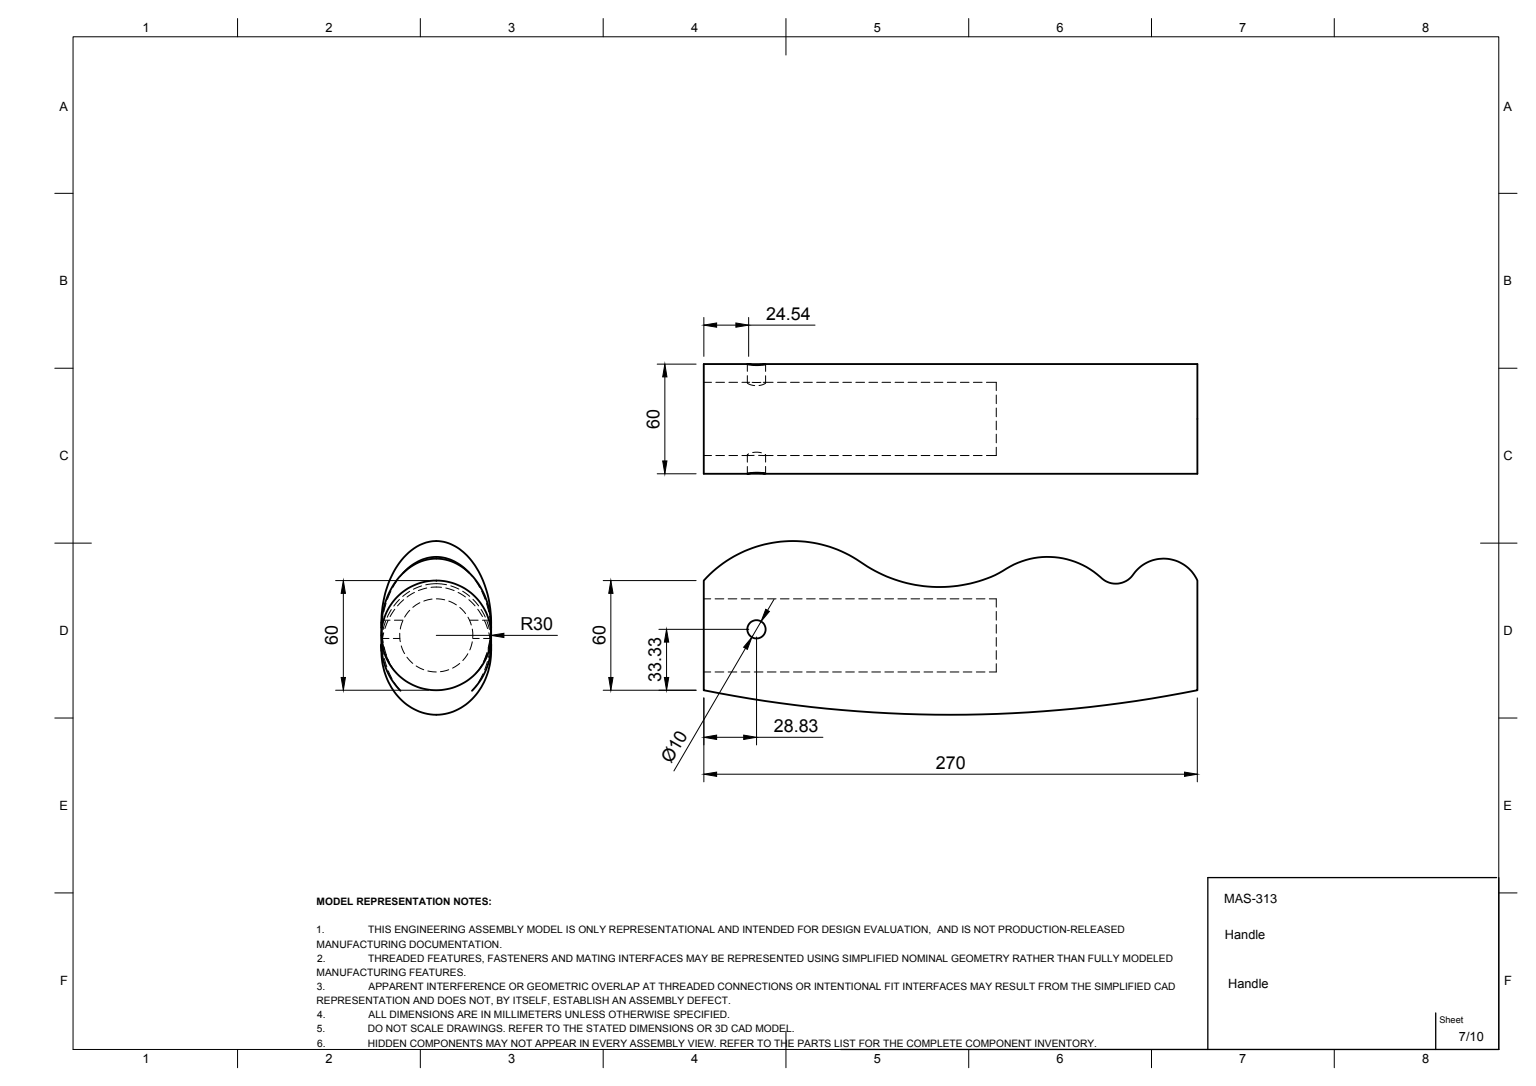
ISO-10303-21;
HEADER;
FILE_DESCRIPTION (('STEP AP214'),
    '1' );
FILE_NAME ('Handle.step',
    '2026-10-06T09:36:00',
    ( '' ),
    ( '' ),
    'SwSTEP 2.0',
    'SolidWorks 2025',
    '' );
FILE_SCHEMA (( 'AUTOMOTIVE_DESIGN' ));
ENDSEC;

DATA;
#4=CARTESIAN_POINT ( 'NONE',  ( -828.8285638327245124, 78.34605190446923473, -105.0145692953451260 ) ) ;
#15=CARTESIAN_POINT ( 'NONE',  ( -795.0000000000070486, 70.44548139156158584, -96.78565065507937959 ) ) ;
#16=CARTESIAN_POINT ( 'NONE',  ( -820.7717470982067880, 82.64484858469236883, -104.6903222377189593 ) ) ;
#19=CARTESIAN_POINT ( 'NONE',  ( -826.0529305544633871, 83.16438776978758085, -144.6472496521801929 ) ) ;
#28=CARTESIAN_POINT ( 'NONE',  ( -976.0610374937461984, 42.74778062430068104, -107.9061927053324155 ) ) ;
#38=CARTESIAN_POINT ( 'NONE',  ( -795.0000000000065938, 109.8950841424301217, -113.1262384684096105 ) ) ;
#41=CARTESIAN_POINT ( 'NONE',  ( -951.5459139781262365, 122.3346817490816676, -136.2353035311979852 ) ) ;
#50=CARTESIAN_POINT ( 'NONE',  ( -954.3284336448712111, 118.5422944683825932, -141.4553492942762318 ) ) ;
#59=CARTESIAN_POINT ( 'NONE',  ( -1046.457602311632627, 98.67849639484583690, -149.7857175106632894 ) ) ;
#60=CARTESIAN_POINT ( 'NONE',  ( -1054.407929976944160, 113.5897173251037628, -130.5712005305405228 ) ) ;
#67=CARTESIAN_POINT ( 'NONE',  ( -1027.708477481189902, 65.70736702952426356, -149.7857175106639431 ) ) ;
#79=CARTESIAN_POINT ( 'NONE',  ( -1062.665377791213132, 57.01990411978262330, -103.3307627799634503 ) ) ;
#82=CARTESIAN_POINT ( 'NONE',  ( -1032.658196452833636, 44.72920460984212809, -126.6442663926291914 ) ) ;
#91=CARTESIAN_POINT ( 'NONE',  ( -953.8433812051914629, 65.95343150956773570, -99.57582448894520155 ) ) ;
#98=CARTESIAN_POINT ( 'NONE',  ( -1054.691024341069351, 108.1159421897237110, -107.9061927053325149 ) ) ;
#104=CARTESIAN_POINT ( 'NONE',  ( -1054.519145619997744, 111.4921997120089401, -113.1262384684101079 ) ) ;
#107=CARTESIAN_POINT ( 'NONE',  ( -1024.848917040341576, 116.4131098345822437, -136.2353035311980420 ) ) ;
#109=CARTESIAN_POINT ( 'NONE',  ( -1045.884592419585942, 115.0579440276405450, -118.7903414690682524 ) ) ;
#113=CARTESIAN_POINT ( 'NONE',  ( -954.7734463792789938, 107.7731650919854758, -149.7857175106632042 ) ) ;
#119=CARTESIAN_POINT ( 'NONE',  ( -1065.000000000006366, 107.1049510380562850, -141.4553492942759192 ) ) ;
#129=CARTESIAN_POINT ( 'NONE',  ( -956.7203770923184720, 58.97922774997713447, -146.0307792196449839 ) ) ;
#137=CARTESIAN_POINT ( 'NONE',  ( -818.1708872189576596, 40.82851623284144438, -103.3307627799635640 ) ) ;
#138=CARTESIAN_POINT ( 'NONE',  ( -823.5000624989293101, 83.67424195610622917, -104.7509713550767287 ) ) ;
#139=CARTESIAN_POINT ( 'NONE',  ( -901.8967518049312275, 57.00804855647886171, -130.5712005305400965 ) ) ;
#140=VERTEX_POINT ( 'NONE', #3194 ) ;
#142=CARTESIAN_POINT ( 'NONE',  ( -825.4378685752795946, 73.92905737501402541, -154.6600603160834169 ) ) ;
#146=CARTESIAN_POINT ( 'NONE',  ( -1021.607260580486013, 54.24386729702176524, -118.7903414690683661 ) ) ;
#155=CARTESIAN_POINT ( 'NONE',  ( -954.3284336448667773, 118.5422944683823800, -107.9061927053323302 ) ) ;
#158=CARTESIAN_POINT ( 'NONE',  ( -1054.519145619990923, 111.4921997120091106, -136.2353035311978999 ) ) ;
#169=CARTESIAN_POINT ( 'NONE',  ( -852.9318753287220716, 113.3383058689776277, -141.4553492942764024 ) ) ;
#178=VERTEX_POINT ( 'NONE', #3366 ) ;
#182=CARTESIAN_POINT ( 'NONE',  ( -956.4793285278399253, 64.87563161486532692, -149.7857175106635452 ) ) ;
#190=CARTESIAN_POINT ( 'NONE',  ( -954.4431216459919369, 51.77564274757662588, -136.2353035311985820 ) ) ;
#194=CARTESIAN_POINT ( 'NONE',  ( -817.4144546772188278, 30.82543593413045713, -113.1262384684093689 ) ) ;
#195=CARTESIAN_POINT ( 'NONE',  ( -822.2163178171820164, 83.41010758653678181, -104.7304854148475499 ) ) ;
#202=CARTESIAN_POINT ( 'NONE',  ( -828.1602791247941013, 76.17169011767150266, -154.6744596958750151 ) ) ;
#207=CARTESIAN_POINT ( 'NONE',  ( -1048.438004920983758, 39.66697241395321782, -122.7172756069793138 ) ) ;
#212=UNCERTAINTY_MEASURE_WITH_UNIT (LENGTH_MEASURE( 1.000000000000000082E-05 ), #7205, 'distance_accuracy_value', 'NONE');
#214=CARTESIAN_POINT ( 'NONE',  ( -951.5459139781289650, 122.3346817490815681, -113.1262384684093263 ) ) ;
#219=CARTESIAN_POINT ( 'NONE',  ( -1061.673215548682720, 86.58918783539685649, -95.06748246948023962 ) ) ;
#220=CARTESIAN_POINT ( 'NONE',  ( -954.0688428831344936, 124.4732772249357282, -130.5712005305405796 ) ) ;
#229=CARTESIAN_POINT ( 'NONE',  ( -1025.044148074459827, 113.2108726315406813, -141.4553492942762318 ) ) ;
#234=CARTESIAN_POINT ( 'NONE',  ( -1010.922847972424620, 120.6260792194949829, -126.6442663926288503 ) ) ;
#237=CARTESIAN_POINT ( 'NONE',  ( -853.1108559448500728, 99.60875591605696400, -149.7857175106632610 ) ) ;
#245=CARTESIAN_POINT ( 'NONE',  ( -956.2104666674752025, 71.56905446038098262, -152.5758913445294809 ) ) ;
#251=CARTESIAN_POINT ( 'NONE',  ( -795.0000000000020464, 52.38665522077208436, -130.5712005305402670 ) ) ;
#252=ORIENTED_EDGE ( 'NONE', *, *, #941, .T. ) ;
#257=CARTESIAN_POINT ( 'NONE',  ( -1014.004070199759440, 54.58258344709550869, -113.1262384684095537 ) ) ;
#259=CARTESIAN_POINT ( 'NONE',  ( -1014.004070199769671, 54.58258344709567922, -136.2353035311988947 ) ) ;
#265=CARTESIAN_POINT ( 'NONE',  ( -976.2351830775012331, 35.86345807843999012, -118.7903414690679824 ) ) ;
#272=CARTESIAN_POINT ( 'NONE',  ( -1031.197907781702725, 107.2697845108577894, -103.3307627799635640 ) ) ;
#279=DIRECTION ( 'NONE',  ( 1.000000000000000000, -1.262554838833776231E-16, 0.000000000000000000 ) ) ;
#282=CARTESIAN_POINT ( 'NONE',  ( -853.3345817150102448, 81.97571759610518427, -95.06748246948041015 ) ) ;
#284=CARTESIAN_POINT ( 'NONE',  ( -823.5047064235034213, 114.4566975831562274, -136.2353035311979284 ) ) ;
#293=CARTESIAN_POINT ( 'NONE',  ( -1037.392967692951970, 114.2240391150264998, -136.2353035311982126 ) ) ;
#300=CARTESIAN_POINT ( 'NONE',  ( -1060.756016675586807, 112.8516620848305934, -124.6807709998040821 ) ) ;
#302=CARTESIAN_POINT ( 'NONE',  ( -1037.550865396555764, 105.7975851359348667, -146.0307792196445860 ) ) ;
#309=CARTESIAN_POINT ( 'NONE',  ( -953.8433812051875975, 65.95343150956774991, -149.7857175106634315 ) ) ;
#313=CARTESIAN_POINT ( 'NONE',  ( -854.0803342822151762, 23.97549884981696167, -130.5712005305403238 ) ) ;
#317=CARTESIAN_POINT ( 'NONE',  ( -1028.454949082212806, 53.01113643315385104, -113.1262384684094400 ) ) ;
#320=CARTESIAN_POINT ( 'NONE',  ( -1038.664246639927342, 43.28664065472985811, -136.2353035311990084 ) ) ;
#326=CARTESIAN_POINT ( 'NONE',  ( -824.4849247483655290, 73.70682285379986354, -154.6506428397234743 ) ) ;
#329=CARTESIAN_POINT ( 'NONE',  ( -1065.000000000003865, 52.00000000000021316, -126.6442663926290493 ) ) ;
#335=CARTESIAN_POINT ( 'NONE',  ( -1061.468168685228193, 92.73456844357777129, -96.78565065507918064 ) ) ;
#341=CIRCLE ( 'NONE', #6268, 30.00000000000021316 ) ;
#345=CARTESIAN_POINT ( 'NONE',  ( -1055.782959745578182, 85.17781532426863578, -95.06748246948041015 ) ) ;
#347=CARTESIAN_POINT ( 'NONE',  ( -1021.743962174751232, 119.2557508373789403, -124.6807709998040110 ) ) ;
#354=CARTESIAN_POINT ( 'NONE',  ( -1048.438004920983303, 39.66697241395321782, -124.6807709998044800 ) ) ;
#360=PLANE ( 'NONE',  #530 ) ;
#361=CARTESIAN_POINT ( 'NONE',  ( -1024.691966601151762, 118.8493250655917564, -126.6442663926291061 ) ) ;
#374=CARTESIAN_POINT ( 'NONE',  ( -827.5978224575839022, 75.37295367873073815, -94.68020981275554959 ) ) ;
#375=( NAMED_UNIT ( * ) SI_UNIT ( $, .STERADIAN. ) SOLID_ANGLE_UNIT ( ) );
#378=CARTESIAN_POINT ( 'NONE',  ( -1062.923339974281134, 49.86928741160674150, -136.2353035311989515 ) ) ;
#382=CARTESIAN_POINT ( 'NONE',  ( -1017.158871447982051, 53.64146012065780411, -122.7172756069791717 ) ) ;
#385=CARTESIAN_POINT ( 'NONE',  ( -822.5313098515729280, 73.83434793536794416, -154.6477719089843390 ) ) ;
#388=CARTESIAN_POINT ( 'NONE',  ( -976.2517683711888594, 35.25052392388814582, -122.7172756069790296 ) ) ;
#393=CARTESIAN_POINT ( 'NONE',  ( -1025.928429817214464, 97.79385104913474436, -96.78565065507955012 ) ) ;
#397=CARTESIAN_POINT ( 'NONE',  ( -795.0000000000002274, 98.77454568802498613, -99.57582448894500260 ) ) ;
#399=CARTESIAN_POINT ( 'NONE',  ( -951.4198147059589701, 125.0824040815807194, -124.6807709998040252 ) ) ;
#410=CARTESIAN_POINT ( 'NONE',  ( -1017.810720698608179, 119.7719591276206046, -126.6442663926290493 ) ) ;
#415=ORIENTED_EDGE ( 'NONE', *, *, #2463, .T. ) ;
#425=CARTESIAN_POINT ( 'NONE',  ( -901.9718911164696920, 59.00785292138922244, -136.2353035311984115 ) ) ;
#430=CARTESIAN_POINT ( 'NONE',  ( -1062.996098538733122, 47.98024286075321498, -118.7903414690683377 ) ) ;
#432=CARTESIAN_POINT ( 'NONE',  ( -824.1522960622456822, 83.67452213711085562, -95.25851046848316628 ) ) ;
#433=CARTESIAN_POINT ( 'NONE',  ( -818.8285638327243987, 78.67432280806558254, -94.73795703228648790 ) ) ;
#437=CARTESIAN_POINT ( 'NONE',  ( -1021.637154595298057, 53.81063926482157456, -126.6442663926291630 ) ) ;
#439=CARTESIAN_POINT ( 'NONE',  ( -818.8285638327238303, 78.67432280806571043, -144.4023295390032899 ) ) ;
#443=CARTESIAN_POINT ( 'NONE',  ( -1031.329434936836833, 101.6864263019767378, -99.57582448894520155 ) ) ;
#453=CARTESIAN_POINT ( 'NONE',  ( -828.7969121913764639, 79.32510138126919230, -154.5423082524717699 ) ) ;
#454=CARTESIAN_POINT ( 'NONE',  ( -1038.158164256576356, 71.32123499372119113, -95.06748246948035330 ) ) ;
#456=CARTESIAN_POINT ( 'NONE',  ( -823.7180591916866206, 117.1502831467254993, -130.5712005305406080 ) ) ;
#464=CARTESIAN_POINT ( 'NONE',  ( -795.0000000000020464, 111.6133447792289530, -118.7903414690682524 ) ) ;
#467=CARTESIAN_POINT ( 'NONE',  ( -795.0000000000048885, 52.00000000000024158, -124.6807709998040821 ) ) ;
#477=CARTESIAN_POINT ( 'NONE',  ( -955.0000000000038654, 102.0000000000005400, -124.6807709998041531 ) ) ;
#480=EDGE_LOOP ( 'NONE', ( #1423, #3316 ) ) ;
#485=CARTESIAN_POINT ( 'NONE',  ( -902.6139906877482417, 77.75433758651681160, -152.5758913445294809 ) ) ;
#486=CARTESIAN_POINT ( 'NONE',  ( -818.9962482452939412, 77.37998253221861944, -144.1405054422210981 ) ) ;
#494=CARTESIAN_POINT ( 'NONE',  ( -1013.844210246968942, 57.79547239392000790, -141.4553492942758908 ) ) ;
#499=CARTESIAN_POINT ( 'NONE',  ( -827.5988398165042099, 81.97491382366440860, -95.05718603569194158 ) ) ;
#506=CARTESIAN_POINT ( 'NONE',  ( -998.0431609429218724, 37.14019503514174403, -126.6442663926292340 ) ) ;
#512=CARTESIAN_POINT ( 'NONE',  ( -974.6181169426257611, 104.3135445892214506, -99.57582448894483207 ) ) ;
#523=CARTESIAN_POINT ( 'NONE',  ( -903.0443340174317655, 90.92133391050421665, -94.48732055948569553 ) ) ;
#526=CARTESIAN_POINT ( 'NONE',  ( -1017.810720698608179, 119.7719591276206046, -126.6442663926290493 ) ) ;
#530=AXIS2_PLACEMENT_3D ( 'NONE', #4144, #3201, #7285 ) ;
#535=CARTESIAN_POINT ( 'NONE',  ( -823.4987033863208126, 83.67412160126858112, -95.25369430085760314 ) ) ;
#538=CARTESIAN_POINT ( 'NONE',  ( -904.2101318206010774, 125.2895275102983419, -122.7172756069790580 ) ) ;
#557=CARTESIAN_POINT ( 'NONE',  ( -824.4876953351460998, 73.70726043279957196, -94.71087641695557124 ) ) ;
#561=CARTESIAN_POINT ( 'NONE',  ( -927.9936929689694125, 74.21188826700395680, -149.7857175106638863 ) ) ;
#570=CARTESIAN_POINT ( 'NONE',  ( -828.7958589970872936, 79.33211491968606310, -94.81972313272032693 ) ) ;
#575=CARTESIAN_POINT ( 'NONE',  ( -955.0000000000038654, 82.00000000000036948, -124.6807709998041673 ) ) ;
#581=CARTESIAN_POINT ( 'NONE',  ( -994.8066578865433485, 80.00401887192406036, -94.48732055948607922 ) ) ;
#592=CARTESIAN_POINT ( 'NONE',  ( -826.3386627754631490, 83.01093823284401196, -154.1821612695491979 ) ) ;
#593=CARTESIAN_POINT ( 'NONE',  ( -902.6139906877451722, 77.75433758651645633, -96.78565065507919485 ) ) ;
#600=CARTESIAN_POINT ( 'NONE',  ( -817.1493800258449482, 27.50875274330016751, -124.6807709998041815 ) ) ;
#602=FACE_OUTER_BOUND ( 'NONE', #11018, .T. ) ;
#603=CARTESIAN_POINT ( 'NONE',  ( -1037.337636019038655, 116.9882293220588991, -122.7172756069792001 ) ) ;
#614=CARTESIAN_POINT ( 'NONE',  ( -1020.082665824768128, 80.34198733739798115, -154.2940595301280950 ) ) ;
#624=ORIENTED_EDGE ( 'NONE', *, *, #2970, .T. ) ;
#625=CARTESIAN_POINT ( 'NONE',  ( -976.0610374937396045, 42.74778062430040393, -141.4553492942756634 ) ) ;
#643=CARTESIAN_POINT ( 'NONE',  ( -1065.000000000006139, 76.10956187831460795, -95.06748246948023962 ) ) ;
#653=CARTESIAN_POINT ( 'NONE',  ( -1012.828629370415570, 79.69572830938430741, -95.06748246948046699 ) ) ;
#668=CARTESIAN_POINT ( 'NONE',  ( -1065.000000000007731, 112.0000000000007105, -122.7172756069790438 ) ) ;
#673=AXIS2_PLACEMENT_3D ( 'NONE', #5309, #8235, #11995 ) ;
#679=CARTESIAN_POINT ( 'NONE',  ( -1061.673215548682947, 86.58918783539726860, -154.2940595301283793 ) ) ;
#684=CARTESIAN_POINT ( 'NONE',  ( -1014.911393615049064, 99.73439156315002663, -152.5758913445290261 ) ) ;
#689=CARTESIAN_POINT ( 'NONE',  ( -1065.000000000003638, 87.89043812168645786, -154.2940595301284361 ) ) ;
#702=CARTESIAN_POINT ( 'NONE',  ( -1065.000000000000682, 52.38665522077219805, -130.5712005305403238 ) ) ;
#717=CARTESIAN_POINT ( 'NONE',  ( -853.5732225365160275, 62.99598188221410311, -95.06748246948041015 ) ) ;
#718=PLANE ( 'NONE',  #10433 ) ;
#732=CARTESIAN_POINT ( 'NONE',  ( -1017.810720698610226, 119.7719591276204625, -122.7172756069789017 ) ) ;
#743=CARTESIAN_POINT ( 'NONE',  ( -994.8066578865465317, 80.00401887192411721, -154.8742214401228523 ) ) ;
#744=CARTESIAN_POINT ( 'NONE',  ( -828.5731535248166892, 77.06390383656801646, -144.0645491675088294 ) ) ;
#747=CARTESIAN_POINT ( 'NONE',  ( -794.9999999999980673, 87.89043812168634418, -154.2940595301278961 ) ) ;
#751=STYLED_ITEM ( 'NONE', ( #7990 ), #8008 ) ;
#754=CARTESIAN_POINT ( 'NONE',  ( -1065.000000000004320, 98.77454568802519930, -149.7857175106631189 ) ) ;
#756=CARTESIAN_POINT ( 'NONE',  ( -1047.392513188124212, 70.23666496464454667, -154.2940595301285214 ) ) ;
#764=CARTESIAN_POINT ( 'NONE',  ( -817.4144546772251942, 30.82543593413060279, -136.2353035311987242 ) ) ;
#776=CARTESIAN_POINT ( 'NONE',  ( -995.4135022096149896, 71.70161378084165449, -95.06748246948046699 ) ) ;
#779=CARTESIAN_POINT ( 'NONE',  ( -820.7807412222841776, 82.64141399635654750, -144.6707558958804043 ) ) ;
#788=CARTESIAN_POINT ( 'NONE',  ( -1062.665377791213132, 57.01990411978262330, -103.3307627799634503 ) ) ;
#803=CARTESIAN_POINT ( 'NONE',  ( -1021.777026427247165, 118.8177985574657924, -118.7903414690675561 ) ) ;
#813=CARTESIAN_POINT ( 'NONE',  ( -1022.719357623492101, 104.5170332807324769, -149.7857175106632610 ) ) ;
#814=CARTESIAN_POINT ( 'NONE',  ( -828.3261744505593924, 76.46613818254142814, -143.9024326026600988 ) ) ;
#823=CARTESIAN_POINT ( 'NONE',  ( -902.8257469293334907, 84.21185948885708683, -154.2940595301280950 ) ) ;
#825=CARTESIAN_POINT ( 'NONE',  ( -1065.000000000003865, 112.0000000000008527, -126.6442663926290493 ) ) ;
#831=CARTESIAN_POINT ( 'NONE',  ( -828.6675604493494802, 77.37337224769281363, -105.2204629476323277 ) ) ;
#842=CARTESIAN_POINT ( 'NONE',  ( -1023.860074334734577, 85.97273905232950142, -94.48732055948609343 ) ) ;
#853=CARTESIAN_POINT ( 'NONE',  ( -902.2382941300801349, 66.55116351576566558, -103.3307627799636066 ) ) ;
#868=CARTESIAN_POINT ( 'NONE',  ( -1018.154501869011938, 114.3413228342526082, -107.9061927053323870 ) ) ;
#873=CARTESIAN_POINT ( 'NONE',  ( -991.5701548301636876, 122.8678427087060214, -124.6807709998040536 ) ) ;
#877=CARTESIAN_POINT ( 'NONE',  ( -1014.632462699976486, 105.5176738732105690, -149.7857175106636589 ) ) ;
#884=CIRCLE ( 'NONE', #7177, 20.00000000000017053 ) ;
#887=CARTESIAN_POINT ( 'NONE',  ( -853.5732225365131853, 62.99598188221416706, -154.2940595301278108 ) ) ;
#896=CARTESIAN_POINT ( 'NONE',  ( -826.3665850287353578, 74.35417337301176133, -106.1988918232332821 ) ) ;
#902=B_SPLINE_CURVE_WITH_KNOTS ( 'NONE', 3,
 ( #9879, #8090, #6047, #354, #5288, #4192, #9064, #5173, #11741, #4138, #6972, #11912, #3432, #2454, #5228, #3196, #7094, #1353, #600, #467 ),
 .UNSPECIFIED., .F., .F.,
 ( 4, 1, 1, 1, 2, 1, 1, 1, 2, 2, 2, 2, 4 ),
 ( 0.000000000000000000, 0.04762575996673557022, 0.07143863995010346635, 0.09525151993347125146, 0.1428772799002068217, 0.1647615404280894369, 0.1757036706920307445, 0.1866458009559719411, 0.2085300614838545563, 0.4016963878702066726, 0.4307237013227157574, 0.6771470142487683308, 1.000000000000000000 ),
 .UNSPECIFIED. ) ;
#910=CARTESIAN_POINT ( 'NONE',  ( -902.2382941300801349, 66.55116351576566558, -103.3307627799636066 ) ) ;
#911=FACE_OUTER_BOUND ( 'NONE', #1496, .T. ) ;
#912=CARTESIAN_POINT ( 'NONE',  ( -901.8785362142587019, 56.55314031071017666, -122.7172756069789017 ) ) ;
#915=VERTEX_POINT ( 'NONE', #5828 ) ;
#919=CARTESIAN_POINT ( 'NONE',  ( -795.0000000000022737, 65.22545431197607968, -99.57582448894522997 ) ) ;
#928=CARTESIAN_POINT ( 'NONE',  ( -1017.963927524554038, 117.4283576114806777, -113.1262384684094968 ) ) ;
#929=VECTOR ( 'NONE', #3107, 1000.000000000000000 ) ;
#935=CARTESIAN_POINT ( 'NONE',  ( -903.0443340174343803, 90.92133391050434454, -154.8742214401225112 ) ) ;
#940=CARTESIAN_POINT ( 'NONE',  ( -1045.864486809339269, 115.5688325305735162, -126.6442663926293477 ) ) ;
#941=EDGE_CURVE ( 'NONE', #178, #9730, #11411, .T. ) ;
#943=CARTESIAN_POINT ( 'NONE',  ( -1061.673215548682947, 86.58918783539726860, -154.2940595301283793 ) ) ;
#948=EDGE_CURVE ( 'NONE', #11949, #8436, #3579, .T. ) ;
#949=CARTESIAN_POINT ( 'NONE',  ( -828.8285638327243987, 78.67432280806561096, -104.9592124606052863 ) ) ;
#950=CARTESIAN_POINT ( 'NONE',  ( -1013.844210246968942, 57.79547239392000790, -141.4553492942758908 ) ) ;
#962=CARTESIAN_POINT ( 'NONE',  ( -1038.401083800584274, 57.54275223462379074, -99.57582448894500260 ) ) ;
#963=CARTESIAN_POINT ( 'NONE',  ( -828.3277261219677712, 80.87986238895041424, -104.7098637035480238 ) ) ;
#964=CARTESIAN_POINT ( 'NONE',  ( -1038.708781889657075, 41.03774456592552156, -130.5712005305402670 ) ) ;
#972=CARTESIAN_POINT ( 'NONE',  ( -956.9243412622536198, 54.10650223846825924, -107.9061927053324439 ) ) ;
#975=ADVANCED_FACE ( 'NONE', ( #911 ), #3858, .T. ) ;
#985=CARTESIAN_POINT ( 'NONE',  ( -1046.261572611724432, 104.4651992465225447, -103.3307627799636208 ) ) ;
#989=CARTESIAN_POINT ( 'NONE',  ( -1045.864486809339724, 115.5688325305733741, -124.6807709998043663 ) ) ;
#995=CARTESIAN_POINT ( 'NONE',  ( -795.0000000000006821, 98.77454568802552615, -149.7857175106634884 ) ) ;
#1001=CARTESIAN_POINT ( 'NONE',  ( -1060.773655115453948, 112.4236047030759238, -130.5712005305406080 ) ) ;
#1002=CARTESIAN_POINT ( 'NONE',  ( -1060.756016675584760, 112.8516620848307355, -126.6442663926292056 ) ) ;
#1021=CARTESIAN_POINT ( 'NONE',  ( -1057.299536696272526, 52.76571712355550403, -103.3307627799637487 ) ) ;
#1025=CARTESIAN_POINT ( 'NONE',  ( -1038.719578313837474, 40.52245044769760085, -126.6442663926297740 ) ) ;
#1035=CARTESIAN_POINT ( 'NONE',  ( -1064.999999999999545, 54.10491585757062438, -113.1262384684097668 ) ) ;
#1041=CARTESIAN_POINT ( 'NONE',  ( -1037.461794897084019, 110.6138330393709879, -107.9061927053326144 ) ) ;
#1051=CARTESIAN_POINT ( 'NONE',  ( -926.8105964072291272, 116.1567348237266515, -103.3307627799635213 ) ) ;
#1053=CARTESIAN_POINT ( 'NONE',  ( -1045.884592419587534, 115.0579440276406871, -130.5712005305406365 ) ) ;
#1056=CARTESIAN_POINT ( 'NONE',  ( -951.4198147059590838, 125.0824040815807194, -122.7172756069790864 ) ) ;
#1060=CARTESIAN_POINT ( 'NONE',  ( -1031.000617048993718, 115.3267894020686697, -136.2353035311981557 ) ) ;
#1067=CARTESIAN_POINT ( 'NONE',  ( -1054.691024341075263, 108.1159421897237962, -141.4553492942763739 ) ) ;
#1074=CARTESIAN_POINT ( 'NONE',  ( -1013.637332661010191, 62.09754518945636903, -146.0307792196449839 ) ) ;
#1082=CARTESIAN_POINT ( 'NONE',  ( -1025.943122242211757, 53.12767954719351593, -130.5712005305404375 ) ) ;
#1088=CARTESIAN_POINT ( 'NONE',  ( -1028.007066121602975, 60.50166182213163069, -103.3307627799636350 ) ) ;
#1091=CARTESIAN_POINT ( 'NONE',  ( -828.0762569670757784, 76.03166466797384260, -154.6764201226847035 ) ) ;
#1097=CARTESIAN_POINT ( 'NONE',  ( -1028.454949082212806, 53.01113643315385104, -113.1262384684094400 ) ) ;
#1103=CARTESIAN_POINT ( 'NONE',  ( -974.3195816561840275, 116.7169707472884141, -107.9061927053320602 ) ) ;
#1110=CARTESIAN_POINT ( 'NONE',  ( -1060.958858734054957, 107.4804882715807963, -107.9061927053325007 ) ) ;
#1115=CARTESIAN_POINT ( 'NONE',  ( -1013.875822516560447, 120.2710389253235519, -124.6807709998039257 ) ) ;
#1119=CARTESIAN_POINT ( 'NONE',  ( -1065.000000000006366, 107.1049510380562850, -141.4553492942759192 ) ) ;
#1127=CARTESIAN_POINT ( 'NONE',  ( -993.0619804577135028, 103.7129695969640579, -149.7857175106631757 ) ) ;
#1137=CARTESIAN_POINT ( 'NONE',  ( -1062.493403002509012, 61.99900353997395541, -149.7857175106634315 ) ) ;
#1142=CARTESIAN_POINT ( 'NONE',  ( -1032.589060384111690, 47.36392975189053800, -136.2353035311989231 ) ) ;
#1148=CARTESIAN_POINT ( 'NONE',  ( -795.0000000000039790, 60.65002596136936575, -103.3307627799632797 ) ) ;
#1149=CARTESIAN_POINT ( 'NONE',  ( -821.6103028745254733, 83.16718542005979486, -104.7144644823257522 ) ) ;
#1150=CARTESIAN_POINT ( 'NONE',  ( -1057.693846703458348, 44.87596864925374973, -136.2353035311986957 ) ) ;
#1158=CARTESIAN_POINT ( 'NONE',  ( -1063.013736978595944, 47.55218547899807646, -122.7172756069792570 ) ) ;
#1163=CARTESIAN_POINT ( 'NONE',  ( -926.5908784743340902, 123.4113341959661767, -113.1262384684093831 ) ) ;
#1171=CARTESIAN_POINT ( 'NONE',  ( -993.6119331254994904, 96.30709745136255151, -96.78565065507915222 ) ) ;
#1175=CARTESIAN_POINT ( 'NONE',  ( -974.1288507787421622, 124.2142274477005657, -122.7172756069789017 ) ) ;
#1182=CARTESIAN_POINT ( 'NONE',  ( -1060.958858734060186, 107.4804882715809526, -141.4553492942761750 ) ) ;
#1185=VERTEX_POINT ( 'NONE', #8357 ) ;
#1186=CARTESIAN_POINT ( 'NONE',  ( -1054.380968608931425, 114.0683136310379524, -124.6807709998043663 ) ) ;
#1188=CARTESIAN_POINT ( 'NONE',  ( -926.9570750291560444, 111.1083136274932031, -149.7857175106636021 ) ) ;
#1197=CARTESIAN_POINT ( 'NONE',  ( -975.5821371384174654, 62.83201726680850641, -152.5758913445291682 ) ) ;
#1205=CARTESIAN_POINT ( 'NONE',  ( -902.0880155070191222, 62.23309906011806447, -107.9061927053322876 ) ) ;
#1211=CARTESIAN_POINT ( 'NONE',  ( -826.8780104611989827, 74.69851342245382853, -154.6772770270139858 ) ) ;
#1214=CARTESIAN_POINT ( 'NONE',  ( -817.2011019090423360, 28.13185037056188875, -118.7903414690680250 ) ) ;
#1217=CARTESIAN_POINT ( 'NONE',  ( -1065.000000000002956, 98.77454568802522772, -99.57582448894488891 ) ) ;
#1224=CARTESIAN_POINT ( 'NONE',  ( -974.9912860506733523, 88.33816101283738931, -95.06748246948018277 ) ) ;
#1226=CARTESIAN_POINT ( 'NONE',  ( -951.4444194419925225, 124.5703232071644209, -130.5712005305403238 ) ) ;
#1227=CARTESIAN_POINT ( 'NONE',  ( -1065.000000000005912, 111.6133447792291093, -130.5712005305407217 ) ) ;
#1232=CARTESIAN_POINT ( 'NONE',  ( -852.8175266017512968, 121.6828083272127685, -122.7172756069790438 ) ) ;
#1242=CARTESIAN_POINT ( 'NONE',  ( -954.0441199534431007, 124.9954171138389398, -126.6442663926288787 ) ) ;
#1244=CARTESIAN_POINT ( 'NONE',  ( -853.0139081111152564, 107.1087209265616735, -146.0307792196445291 ) ) ;
#1251=CARTESIAN_POINT ( 'NONE',  ( -1038.283672687649414, 64.16172732404312740, -152.5758913445294240 ) ) ;
#1259=CARTESIAN_POINT ( 'NONE',  ( -954.5446161821273563, 49.54000128949434867, -118.7903414690681103 ) ) ;
#1266=CARTESIAN_POINT ( 'NONE',  ( -825.8920934164954133, 74.11705420691500024, -154.6655862438749409 ) ) ;
#1272=CARTESIAN_POINT ( 'NONE',  ( -795.0000000000047748, 52.00000000000024158, -122.7172756069790154 ) ) ;
#1278=CARTESIAN_POINT ( 'NONE',  ( -1061.276350651669873, 98.40484402385480678, -99.57582448894525839 ) ) ;
#1287=CARTESIAN_POINT ( 'NONE',  ( -1015.209561144954137, 93.46821065761379543, -95.06748246948018277 ) ) ;
#1289=CARTESIAN_POINT ( 'NONE',  ( -823.7180591916866206, 117.1502831467254993, -130.5712005305406080 ) ) ;
#1293=CARTESIAN_POINT ( 'NONE',  ( -852.8274699693115508, 120.9962006285026774, -118.7903414690677124 ) ) ;
#1303=FACE_BOUND ( 'NONE', #6936, .T. ) ;
#1305=CARTESIAN_POINT ( 'NONE',  ( -1011.662592067699165, 105.4443429699074244, -149.7857175106632326 ) ) ;
#1311=CARTESIAN_POINT ( 'NONE',  ( -823.4970567115327640, 73.67398878492954850, -106.4962298347511620 ) ) ;
#1315=CARTESIAN_POINT ( 'NONE',  ( -820.0645691041015652, 75.36693519558788523, -94.68454641646253833 ) ) ;
#1320=CARTESIAN_POINT ( 'NONE',  ( -854.0393178910176175, 26.93106345811105840, -113.1262384684097100 ) ) ;
#1331=CARTESIAN_POINT ( 'NONE',  ( -954.4431216459856842, 51.77564274757639140, -113.1262384684095537 ) ) ;
#1337=CARTESIAN_POINT ( 'NONE',  ( -954.5323978148114747, 113.6695689568732206, -103.3307627799632513 ) ) ;
#1341=COLOUR_RGB ( '', 0.08235294, 0.09019608, 0.10196078) ;
#1343=CARTESIAN_POINT ( 'NONE',  ( -1025.928429817214464, 97.79385104913474436, -96.78565065507955012 ) ) ;
#1346=CARTESIAN_POINT ( 'NONE',  ( -823.7697810748826441, 117.7733807739869292, -126.6442663926291914 ) ) ;
#1350=CARTESIAN_POINT ( 'NONE',  ( -1037.392967692957200, 114.2240391150264855, -113.1262384684098805 ) ) ;
#1353=CARTESIAN_POINT ( 'NONE',  ( -854.0902776497798641, 23.28889115110666808, -124.6807709998044800 ) ) ;
#1359=CARTESIAN_POINT ( 'NONE',  ( -1065.000000000006594, 112.0000000000007105, -124.6807709998041531 ) ) ;
#1367=CARTESIAN_POINT ( 'NONE',  ( -1019.723937646960849, 86.79129919622100431, -154.8742214401232502 ) ) ;
#1370=CARTESIAN_POINT ( 'NONE',  ( -822.5396358769451126, 73.84052889928489094, -94.71353457946125332 ) ) ;
#1375=CARTESIAN_POINT ( 'NONE',  ( -1038.401083800579045, 57.54275223462362021, -149.7857175106632326 ) ) ;
#1379=CARTESIAN_POINT ( 'NONE',  ( -976.2517683711888594, 35.25052392388814582, -122.7172756069790296 ) ) ;
#1384=ORIENTED_EDGE ( 'NONE', *, *, #7764, .F. ) ;
#1391=CARTESIAN_POINT ( 'NONE',  ( -1065.000000000004093, 93.55451860843899681, -96.78565065507908116 ) ) ;
#1399=CARTESIAN_POINT ( 'NONE',  ( -820.0633694947518961, 81.98028010177233682, -154.3548397009152779 ) ) ;
#1400=CARTESIAN_POINT ( 'NONE',  ( -1037.899050076301137, 86.18944477603540122, -95.06748246948046699 ) ) ;
#1402=CARTESIAN_POINT ( 'NONE',  ( -904.1919162299276422, 124.8346192645298487, -130.5712005305403807 ) ) ;
#1403=CARTESIAN_POINT ( 'NONE',  ( -1030.931480980267906, 117.9615145441170654, -124.6807709998043521 ) ) ;
#1416=CARTESIAN_POINT ( 'NONE',  ( -852.8175266017517515, 121.6828083272129106, -126.6442663926292624 ) ) ;
#1423=ORIENTED_EDGE ( 'NONE', *, *, #948, .F. ) ;
#1434=CARTESIAN_POINT ( 'NONE',  ( -954.0832773815118344, 60.15510303592687080, -146.0307792196447565 ) ) ;
#1437=CARTESIAN_POINT ( 'NONE',  ( -998.0431609429222135, 37.14019503514177956, -122.7172756069792854 ) ) ;
#1444=CARTESIAN_POINT ( 'NONE',  ( -1054.913455627178109, 103.6024512377076263, -103.3307627799635640 ) ) ;
#1459=CARTESIAN_POINT ( 'NONE',  ( -955.0000000000038654, 102.0000000000005400, -124.6807709998041531 ) ) ;
#1460=CARTESIAN_POINT ( 'NONE',  ( -828.8285638327243987, 78.67432280806596623, -144.4023295390031194 ) ) ;
#1465=CARTESIAN_POINT ( 'NONE',  ( -823.7180591916842332, 117.1502831467252150, -118.7903414690680535 ) ) ;
#1472=CARTESIAN_POINT ( 'NONE',  ( -822.5268906875147650, 83.51316246527650833, -95.22287600579254274 ) ) ;
#1474=CARTESIAN_POINT ( 'NONE',  ( -1017.810720698609543, 119.7719591276204625, -124.6807709998040679 ) ) ;
#1485=AXIS2_PLACEMENT_3D ( 'NONE', #575, #1758, #3529 ) ;
#1488=CARTESIAN_POINT ( 'NONE',  ( -794.9999999999992042, 76.10956187831466480, -154.2940595301278393 ) ) ;
#1494=CARTESIAN_POINT ( 'NONE',  ( -1065.000000000000909, 56.89504896194504369, -141.4553492942757771 ) ) ;
#1496=EDGE_LOOP ( 'NONE', ( #3127, #7189 ) ) ;
#1509=CARTESIAN_POINT ( 'NONE',  ( -903.2629211055218548, 97.63080833215146015, -95.06748246947979908 ) ) ;
#1518=CARTESIAN_POINT ( 'NONE',  ( -1019.723937646958007, 86.79129919622097589, -94.48732055948626396 ) ) ;
#1521=CARTESIAN_POINT ( 'NONE',  ( -954.0441199534440102, 124.9954171138387977, -124.6807709998039115 ) ) ;
#1534=CARTESIAN_POINT ( 'NONE',  ( -926.5138833012647410, 125.7648744980332225, -124.6807709998040394 ) ) ;
#1549=CARTESIAN_POINT ( 'NONE',  ( -828.8285638327240576, 78.67432280806576728, -94.77914401073080342 ) ) ;
#1552=CARTESIAN_POINT ( 'NONE',  ( -1038.595419435783924, 46.89684673038589580, -141.4553492942758623 ) ) ;
#1566=ORIENTED_EDGE ( 'NONE', *, *, #7764, .T. ) ;
#1567=CARTESIAN_POINT ( 'NONE',  ( -928.4368846968637854, 59.55532739646334051, -126.6442663926292056 ) ) ;
#1571=CARTESIAN_POINT ( 'NONE',  ( -819.4913475613807350, 81.18356759358016461, -154.4422483361309446 ) ) ;
#1572=CARTESIAN_POINT ( 'NONE',  ( -1047.151245865161172, 77.61790247226321071, -94.48732055948626396 ) ) ;
#1581=CARTESIAN_POINT ( 'NONE',  ( -927.4753839990671622, 92.66010094724835255, -94.48732055948569553 ) ) ;
#1588=CARTESIAN_POINT ( 'NONE',  ( -818.8285638327251945, 78.67432280806566780, -154.6235849673217899 ) ) ;
#1590=CARTESIAN_POINT ( 'NONE',  ( -795.0000000000047748, 112.0000000000007532, -124.6807709998042384 ) ) ;
#1592=ADVANCED_FACE ( 'NONE', ( #2099, #9451 ), #10284, .T. ) ;
#1601=CARTESIAN_POINT ( 'NONE',  ( -1046.909978542192675, 84.99913997988247161, -154.2940595301286919 ) ) ;
#1602=CARTESIAN_POINT ( 'NONE',  ( -828.7636281597818879, 77.85463023298339635, -144.2471423470013576 ) ) ;
#1605=CARTESIAN_POINT ( 'NONE',  ( -1012.226803665787770, 93.06815595962714838, -154.2940595301283224 ) ) ;
#1612=CARTESIAN_POINT ( 'NONE',  ( -1016.652307257396728, 63.31440937415337800, -146.0307792196454102 ) ) ;
#1616=B_SPLINE_CURVE_WITH_KNOTS ( 'NONE', 3,
 ( #6872, #8786, #8954, #10641, #486, #2180, #7983, #5942, #11640, #7925, #10697, #11695, #2292, #11813, #6061, #6302, #6247, #1667, #7235, #8300, #7172, #1741, #8233, #11000, #9079, #9208, #3329, #5429, #8103, #10872, #4390, #9141, #3508, #2528, #814, #744, #7109, #1602, #2408, #2653, #4333, #2471 ),
 .UNSPECIFIED., .F., .F.,
 ( 4, 2, 2, 2, 2, 2, 2, 2, 2, 2, 2, 2, 2, 2, 2, 2, 2, 2, 2, 2, 4 ),
 ( 0.000000000000000000, 0.0009975002171434010391, 0.001496250325715081392, 0.001995000434286762180, 0.002992500651430000155, 0.003990000868573238997, 0.004987501085716477406, 0.005486251194287953062, 0.005985001302859429585, 0.006982501520002396510, 0.007980001737145364302, 0.008478751845717013430, 0.008977501954288664293, 0.009975002171431972958, 0.01097250238857527989, 0.01197000260571858508, 0.01296750282286189375, 0.01396500304000520068, 0.01496250325714850934, 0.01546125336572015327, 0.01596000347429179719 ),
 .UNSPECIFIED. ) ;
#1628=CARTESIAN_POINT ( 'NONE',  ( -1057.805062346506702, 42.77845103615944566, -130.5712005305404944 ) ) ;
#1632=CARTESIAN_POINT ( 'NONE',  ( -952.9945178120592573, 87.05516224832913963, -94.48732055948602238 ) ) ;
#1634=ADVANCED_FACE ( 'NONE', ( #1303, #5056 ), #11683, .T. ) ;
#1641=CARTESIAN_POINT ( 'NONE',  ( -975.1903095749676140, 79.73237568579435219, -94.48732055948607922 ) ) ;
#1643=FACE_OUTER_BOUND ( 'NONE', #480, .T. ) ;
#1655=CARTESIAN_POINT ( 'NONE',  ( -1030.931480980269043, 117.9615145441170654, -122.7172756069790722 ) ) ;
#1656=DIRECTION ( 'NONE',  ( 0.000000000000000000, -1.000000000000000000, -4.625929269271452387E-16 ) ) ;
#1666=CARTESIAN_POINT ( 'NONE',  ( -1046.457602311632627, 98.67849639484583690, -149.7857175106632894 ) ) ;
#1667=CARTESIAN_POINT ( 'NONE',  ( -822.1849787629572575, 73.94083650471947067, -142.9856651621330457 ) ) ;
#1672=CARTESIAN_POINT ( 'NONE',  ( -994.1998135634695473, 88.30642396300672203, -154.2940595301282656 ) ) ;
#1679=CARTESIAN_POINT ( 'NONE',  ( -927.8303129675907712, 79.95948428978974221, -152.5758913445291682 ) ) ;
#1696=CARTESIAN_POINT ( 'NONE',  ( -818.8285638327251945, 78.67432280806566780, -154.6235849673217899 ) ) ;
#1698=CARTESIAN_POINT ( 'NONE',  ( -795.0000000000004547, 76.10956187831470743, -95.06748246948018277 ) ) ;
#1700=CARTESIAN_POINT ( 'NONE',  ( -1065.000000000003865, 52.00000000000021316, -126.6442663926290493 ) ) ;
#1710=CARTESIAN_POINT ( 'NONE',  ( -952.9945178120592573, 87.05516224832913963, -94.48732055948602238 ) ) ;
#1711=FACE_BOUND ( 'NONE', #6862, .T. ) ;
#1729=CARTESIAN_POINT ( 'NONE',  ( -991.5701548301638013, 122.8678427087060214, -122.7172756069787170 ) ) ;
#1740=CARTESIAN_POINT ( 'NONE',  ( -1065.000000000003638, 87.89043812168645786, -154.2940595301284361 ) ) ;
#1741=CARTESIAN_POINT ( 'NONE',  ( -823.9892610140105944, 73.67413949648602056, -142.8653811665928686 ) ) ;
#1748=CARTESIAN_POINT ( 'NONE',  ( -1056.430032577873362, 71.19035303699479300, -154.2940595301283793 ) ) ;
#1758=DIRECTION ( 'NONE',  ( 1.000000000000000000, -1.262554838833776231E-16, 0.000000000000000000 ) ) ;
#1765=CARTESIAN_POINT ( 'NONE',  ( -821.0802431487063586, 81.36881375820571805, -95.06748246948008330 ) ) ;
#1768=CARTESIAN_POINT ( 'NONE',  ( -901.8785362142589292, 56.55314031071017666, -126.6442663926291061 ) ) ;
#1769=CARTESIAN_POINT ( 'NONE',  ( -826.8836092318815645, 82.64591421739883970, -144.6711677827317430 ) ) ;
#1775=CARTESIAN_POINT ( 'NONE',  ( -818.6751755801135459, 47.70925804672316417, -99.57582448894514471 ) ) ;
#1778=DIRECTION ( 'NONE',  ( 0.000000000000000000, 1.000000000000000000, 6.938893903907169213E-16 ) ) ;
#1780=ADVANCED_FACE ( 'NONE', ( #11041 ), #6470, .F. ) ;
#1797=CARTESIAN_POINT ( 'NONE',  ( -1061.468168685229102, 92.73456844357778550, -152.5758913445291398 ) ) ;
#1808=CARTESIAN_POINT ( 'NONE',  ( -1015.517346982278013, 86.95624952299075971, -154.8742214401231649 ) ) ;
#1809=CARTESIAN_POINT ( 'NONE',  ( -795.0000000000040927, 111.6133447792292088, -130.5712005305403522 ) ) ;
#1823=DIRECTION ( 'NONE',  ( 1.000000000000000000, 0.000000000000000000, 0.000000000000000000 ) ) ;
#1827=CARTESIAN_POINT ( 'NONE',  ( -954.0832773815070595, 60.15510303592672869, -103.3307627799632513 ) ) ;
#1836=CARTESIAN_POINT ( 'NONE',  ( -1062.810894920125520, 52.92335929224832825, -107.9061927053327139 ) ) ;
#1837=DIRECTION ( 'NONE',  ( 0.000000000000000000, 5.522905491341382306E-16, 1.000000000000000000 ) ) ;
#1840=CARTESIAN_POINT ( 'NONE',  ( -926.6866529578969676, 120.3119365386820192, -107.9061927053322734 ) ) ;
#1850=CARTESIAN_POINT ( 'NONE',  ( -795.0000000000002274, 107.1049510380560719, -107.9061927053326002 ) ) ;
#1859=CARTESIAN_POINT ( 'NONE',  ( -794.9999999999980673, 87.89043812168634418, -154.2940595301278961 ) ) ;
#1862=CARTESIAN_POINT ( 'NONE',  ( -821.0802431487052218, 81.36881375820613016, -154.2940595301280382 ) ) ;
#1869=CARTESIAN_POINT ( 'NONE',  ( -795.0000000000094360, 82.00000000000081002, -154.8742214401225397 ) ) ;
#1875=CARTESIAN_POINT ( 'NONE',  ( -828.5766943389870676, 80.27470094935115696, -144.6085013259159098 ) ) ;
#1878=CARTESIAN_POINT ( 'NONE',  ( -1025.595947590964442, 58.17469240935094632, -141.4553492942760329 ) ) ;
#1883=DIRECTION ( 'NONE',  ( 0.000000000000000000, -1.000000000000000000, -4.625929269271452387E-16 ) ) ;
#1890=CARTESIAN_POINT ( 'NONE',  ( -1020.755281158177013, 68.40999151392674094, -99.57582448894541471 ) ) ;
#1891=CARTESIAN_POINT ( 'NONE',  ( -820.5194676126043305, 82.43685310047874282, -104.6842045117120534 ) ) ;
#1892=CARTESIAN_POINT ( 'NONE',  ( -819.8521517457915024, 81.72352651608187557, -144.6807563939349848 ) ) ;
#1899=CARTESIAN_POINT ( 'NONE',  ( -1065.000000000007049, 56.89504896194527106, -107.9061927053324581 ) ) ;
#1908=CARTESIAN_POINT ( 'NONE',  ( -926.5908784743340902, 123.4113341959661767, -113.1262384684093831 ) ) ;
#1918=CARTESIAN_POINT ( 'NONE',  ( -1037.550865396555764, 105.7975851359348667, -146.0307792196445860 ) ) ;
#1926=CARTESIAN_POINT ( 'NONE',  ( -1046.909978542192675, 84.99913997988247161, -154.2940595301286919 ) ) ;
#1933=CARTESIAN_POINT ( 'NONE',  ( -827.8097080315070571, 81.71711720835189396, -144.6806456489627806 ) ) ;
#1947=CARTESIAN_POINT ( 'NONE',  ( -927.8303129675875880, 79.95948428978934430, -96.78565065507952170 ) ) ;
#1950=CARTESIAN_POINT ( 'NONE',  ( -1014.107508992743988, 52.59077491224116585, -130.5712005305404944 ) ) ;
#1951=CARTESIAN_POINT ( 'NONE',  ( -821.3235167497211933, 83.01396457509433446, -144.6558853884952214 ) ) ;
#1958=DIRECTION ( 'NONE',  ( 1.000000000000000000, 0.000000000000000000, 0.000000000000000000 ) ) ;
#1960=CARTESIAN_POINT ( 'NONE',  ( -817.7441816825951264, 35.12288937987695903, -107.9061927053327281 ) ) ;
#1975=CARTESIAN_POINT ( 'NONE',  ( -954.5323978148114747, 113.6695689568732206, -103.3307627799632513 ) ) ;
#1979=CARTESIAN_POINT ( 'NONE',  ( -1037.337636019038655, 116.9882293220588991, -122.7172756069792001 ) ) ;
#1983=CARTESIAN_POINT ( 'NONE',  ( -1018.154501869017849, 114.3413228342528214, -141.4553492942762887 ) ) ;
#1989=CARTESIAN_POINT ( 'NONE',  ( -926.8105964072267398, 116.1567348237267083, -146.0307792196442733 ) ) ;
#1996=CARTESIAN_POINT ( 'NONE',  ( -927.9936929689694125, 74.21188826700395680, -149.7857175106638863 ) ) ;
#2004=CARTESIAN_POINT ( 'NONE',  ( -1065.000000000007049, 54.10491585757074517, -136.2353035311986389 ) ) ;
#2008=CARTESIAN_POINT ( 'NONE',  ( -956.2104666674714508, 71.56905446038054208, -96.78565065507946485 ) ) ;
#2009=CARTESIAN_POINT ( 'NONE',  ( -827.6025323198989554, 81.97067649012242896, -104.6794282814521750 ) ) ;
#2012=CARTESIAN_POINT ( 'NONE',  ( -1011.051362836436624, 118.1813008219153716, -136.2353035311982126 ) ) ;
#2017=CARTESIAN_POINT ( 'NONE',  ( -795.0000000000039790, 60.65002596136936575, -103.3307627799632797 ) ) ;
#2025=ORIENTED_EDGE ( 'NONE', *, *, #8381, .F. ) ;
#2028=CARTESIAN_POINT ( 'NONE',  ( -1014.007272717921069, 117.9006809476441049, -113.1262384684097526 ) ) ;
#2038=CARTESIAN_POINT ( 'NONE',  ( -974.6181169426273527, 104.3135445892218200, -149.7857175106634884 ) ) ;
#2044=CARTESIAN_POINT ( 'NONE',  ( -1031.197907781699314, 107.2697845108579173, -146.0307792196445291 ) ) ;
#2051=CARTESIAN_POINT ( 'NONE',  ( -819.8422515189698743, 75.63891865958764527, -105.7172146583293681 ) ) ;
#2053=CARTESIAN_POINT ( 'NONE',  ( -1016.652307257396728, 63.31440937415337800, -146.0307792196454102 ) ) ;
#2062=CARTESIAN_POINT ( 'NONE',  ( -954.5446161821218993, 49.54000128949421367, -130.5712005305404091 ) ) ;
#2065=EDGE_CURVE ( 'NONE', #5919, #11269, #7707, .T. ) ;
#2070=CARTESIAN_POINT ( 'NONE',  ( -975.7625022073081027, 55.15120678236761620, -99.57582448894500260 ) ) ;
#2072=CARTESIAN_POINT ( 'NONE',  ( -1065.000000000007049, 54.10491585757074517, -136.2353035311986389 ) ) ;
#2074=CARTESIAN_POINT ( 'NONE',  ( -818.8285638327238303, 78.67432280806571043, -144.4023295390032899 ) ) ;
#2084=CARTESIAN_POINT ( 'NONE',  ( -1065.000000000004093, 52.00000000000021316, -122.7172756069792854 ) ) ;
#2096=CARTESIAN_POINT ( 'NONE',  ( -1065.000000000005230, 87.89043812168627312, -95.06748246948058068 ) ) ;
#2098=CARTESIAN_POINT ( 'NONE',  ( -1013.901471336339000, 119.8325901201404804, -130.5712005305404944 ) ) ;
#2099=FACE_OUTER_BOUND ( 'NONE', #7879, .T. ) ;
#2102=EDGE_CURVE ( 'NONE', #10282, #8579, #884, .T. ) ;
#2106=CARTESIAN_POINT ( 'NONE',  ( -1045.967528061855091, 112.8272211019271225, -136.2353035311980705 ) ) ;
#2110=CARTESIAN_POINT ( 'NONE',  ( -822.2439855206093853, 97.57287547056431265, -149.7857175106634600 ) ) ;
#2117=CARTESIAN_POINT ( 'NONE',  ( -1020.430183747032629, 74.13649791779326392, -152.5758913445297651 ) ) ;
#2131=CARTESIAN_POINT ( 'NONE',  ( -997.7839878466058963, 40.27522178589197921, -113.1262384684093547 ) ) ;
#2132=CARTESIAN_POINT ( 'NONE',  ( -822.5306970061956235, 83.50573423571573528, -104.7374748144106462 ) ) ;
#2134=CARTESIAN_POINT ( 'NONE',  ( -818.8285638327239440, 79.00056486032038094, -144.4573442453753103 ) ) ;
#2140=CARTESIAN_POINT ( 'NONE',  ( -1021.637154595298057, 53.81063926482157456, -122.7172756069792285 ) ) ;
#2144=CARTESIAN_POINT ( 'NONE',  ( -853.0139081111171890, 107.1087209265617020, -103.3307627799635355 ) ) ;
#2151=CARTESIAN_POINT ( 'NONE',  ( -1061.276350651669873, 98.40484402385480678, -99.57582448894525839 ) ) ;
#2155=CARTESIAN_POINT ( 'NONE',  ( -1014.007272717915953, 117.9006809476442896, -136.2353035311982126 ) ) ;
#2159=CARTESIAN_POINT ( 'NONE',  ( -1010.922847972426780, 120.6260792194948550, -122.7172756069790296 ) ) ;
#2164=LINE ( 'NONE', #9694, #10636 ) ;
#2166=CARTESIAN_POINT ( 'NONE',  ( -1017.963927524549604, 117.4283576114808625, -136.2353035311979284 ) ) ;
#2171=CARTESIAN_POINT ( 'NONE',  ( -1010.922847972425529, 120.6260792194948550, -124.6807709998039542 ) ) ;
#2179=CARTESIAN_POINT ( 'NONE',  ( -975.7625022073049195, 55.15120678236734619, -149.7857175106636589 ) ) ;
#2180=CARTESIAN_POINT ( 'NONE',  ( -819.0908526083459265, 77.06787236046235989, -144.0637517540457679 ) ) ;
#2188=CARTESIAN_POINT ( 'NONE',  ( -817.7441816825951264, 35.12288937987695903, -107.9061927053327281 ) ) ;
#2197=CARTESIAN_POINT ( 'NONE',  ( -928.4368846968627622, 59.55532739646334051, -122.7172756069790154 ) ) ;
#2201=CARTESIAN_POINT ( 'NONE',  ( -1011.662592067698938, 105.4443429699071828, -99.57582448894505944 ) ) ;
#2206=CARTESIAN_POINT ( 'NONE',  ( -927.1204550305436669, 105.3607176047075029, -96.78565065507918064 ) ) ;
#2208=CARTESIAN_POINT ( 'NONE',  ( -904.1919162299276422, 124.8346192645298487, -130.5712005305403807 ) ) ;
#2225=CARTESIAN_POINT ( 'NONE',  ( -954.3284336448712111, 118.5422944683825932, -141.4553492942762318 ) ) ;
#2232=CARTESIAN_POINT ( 'NONE',  ( -823.1660337641055776, 73.70728137675567382, -106.4808805636502740 ) ) ;
#2233=CARTESIAN_POINT ( 'NONE',  ( -1025.323167507848893, 62.35287014669186334, -146.0307792196450691 ) ) ;
#2238=B_SPLINE_CURVE_WITH_KNOTS ( 'NONE', 3,
 ( #4308, #3360, #453, #8079, #3483, #11901, #11848, #6224, #6279, #5279, #9054, #592, #4366, #8269, #3419, #4429, #2329, #12027, #7208, #2502, #10049, #8205, #11964, #11035, #2564, #10108, #7021, #1399, #10389, #1571, #7385, #6269, #11956, #5392, #6391, #1696 ),
 .UNSPECIFIED., .F., .F.,
 ( 4, 2, 2, 2, 2, 2, 2, 2, 2, 2, 2, 2, 2, 2, 2, 2, 2, 4 ),
 ( 0.01563545586487890063, 0.01661450767168204737, 0.01759355947848519064, 0.01857261128528833738, 0.01955166309209148412, 0.02053071489889463086, 0.02150976670569777413, 0.02248881851250092087, 0.02346787031930406414, 0.02444692212610721088, 0.02493644802950895079, 0.02542597393291068722, 0.02640502573971446193, 0.02738407754651823664, 0.02836312935332201135, 0.02934218116012578953, 0.03032123296692956424, 0.03130028477373333895 ),
 .UNSPECIFIED. ) ;
#2239=CARTESIAN_POINT ( 'NONE',  ( -828.5735791249488784, 77.06472017290390397, -94.70715242654415533 ) ) ;
#2242=CARTESIAN_POINT ( 'NONE',  ( -997.9925905826634107, 37.72784750336339954, -130.5712005305403238 ) ) ;
#2246=CARTESIAN_POINT ( 'NONE',  ( -1016.863910020555409, 59.13213530333446499, -107.9061927053325576 ) ) ;
#2248=ORIENTED_EDGE ( 'NONE', *, *, #7195, .F. ) ;
#2256=CARTESIAN_POINT ( 'NONE',  ( -1038.708781889661850, 41.03774456592562103, -118.7903414690682240 ) ) ;
#2262=CARTESIAN_POINT ( 'NONE',  ( -1022.396981161626059, 109.5926079579672319, -103.3307627799638482 ) ) ;
#2269=CARTESIAN_POINT ( 'NONE',  ( -853.1108559448483675, 99.60875591605646662, -99.57582448894477523 ) ) ;
#2271=CARTESIAN_POINT ( 'NONE',  ( -954.0441199534431007, 124.9954171138389398, -126.6442663926288787 ) ) ;
#2291=CARTESIAN_POINT ( 'NONE',  ( -1026.651933061287082, 84.71212313386841686, -154.8742214401230228 ) ) ;
#2292=CARTESIAN_POINT ( 'NONE',  ( -820.7495229154759500, 74.72132575352402739, -143.3103177350649844 ) ) ;
#2301=CARTESIAN_POINT ( 'NONE',  ( -956.7203770923184720, 58.97922774997713447, -146.0307792196449839 ) ) ;
#2307=CARTESIAN_POINT ( 'NONE',  ( -1014.132585063772353, 52.13780504951625261, -122.7172756069792428 ) ) ;
#2312=CARTESIAN_POINT ( 'NONE',  ( -823.1766404291720391, 73.70610174456017205, -154.6458666179561590 ) ) ;
#2313=ORIENTED_EDGE ( 'NONE', *, *, #4480, .F. ) ;
#2323=CARTESIAN_POINT ( 'NONE',  ( -993.6119331254994904, 96.30709745136255151, -96.78565065507915222 ) ) ;
#2329=CARTESIAN_POINT ( 'NONE',  ( -824.1625816070830979, 83.67410183576217264, -154.1030193367455468 ) ) ;
#2330=CARTESIAN_POINT ( 'NONE',  ( -1055.176328965296989, 98.13059730676610570, -99.57582448894517313 ) ) ;
#2332=CARTESIAN_POINT ( 'NONE',  ( -1010.922847972425529, 120.6260792194948550, -124.6807709998039542 ) ) ;
#2338=CARTESIAN_POINT ( 'NONE',  ( -1021.913416468816195, 116.8879375517085890, -113.1262384684096673 ) ) ;
#2344=CARTESIAN_POINT ( 'NONE',  ( -819.0912165218314840, 80.28194760164100785, -94.83880827393758750 ) ) ;
#2349=CARTESIAN_POINT ( 'NONE',  ( -926.5138833012656505, 125.7648744980332225, -126.6442663926294330 ) ) ;
#2358=CARTESIAN_POINT ( 'NONE',  ( -1062.096538105497302, 73.81465972843197676, -154.2940595301284930 ) ) ;
#2361=CARTESIAN_POINT ( 'NONE',  ( -822.2256338312696471, 73.93538682641413118, -94.71157759278341359 ) ) ;
#2365=CARTESIAN_POINT ( 'NONE',  ( -1016.863910020547223, 59.13213530333427315, -141.4553492942757487 ) ) ;
#2369=CARTESIAN_POINT ( 'NONE',  ( -817.2011019090423360, 28.13185037056188875, -118.7903414690680250 ) ) ;
#2376=CARTESIAN_POINT ( 'NONE',  ( -1061.673215548682720, 86.58918783539685649, -95.06748246948023962 ) ) ;
#2386=CARTESIAN_POINT ( 'NONE',  ( -902.8257469293350823, 84.21185948885704420, -95.06748246948052383 ) ) ;
#2388=CARTESIAN_POINT ( 'NONE',  ( -1060.756016675584760, 112.8516620848307355, -126.6442663926292056 ) ) ;
#2395=ORIENTED_EDGE ( 'NONE', *, *, #3479, .F. ) ;
#2397=CARTESIAN_POINT ( 'NONE',  ( -852.8274699693115508, 120.9962006285026774, -118.7903414690677124 ) ) ;
#2407=CARTESIAN_POINT ( 'NONE',  ( -1027.019426772554198, 78.04595964998465263, -154.2940595301285782 ) ) ;
#2408=CARTESIAN_POINT ( 'NONE',  ( -828.7881391349023943, 78.01879388416071492, -144.2812265043196760 ) ) ;
#2411=CARTESIAN_POINT ( 'NONE',  ( -822.6980360219018849, 73.80108637340964606, -94.71426656347418316 ) ) ;
#2413=CARTESIAN_POINT ( 'NONE',  ( -1025.595947590964442, 58.17469240935094632, -141.4553492942760329 ) ) ;
#2414=AXIS2_PLACEMENT_3D ( 'NONE', #2699, #8405, #12169 ) ;
#2424=EDGE_CURVE ( 'NONE', #4637, #11949, #8947, .T. ) ;
#2430=CARTESIAN_POINT ( 'NONE',  ( -1056.106496161727136, 78.18408418063160070, -94.48732055948630659 ) ) ;
#2442=CARTESIAN_POINT ( 'NONE',  ( -1015.825132819593136, 80.44428838836749662, -95.06748246948035330 ) ) ;
#2450=CARTESIAN_POINT ( 'NONE',  ( -1014.007272717921069, 117.9006809476441049, -113.1262384684097526 ) ) ;
#2454=CARTESIAN_POINT ( 'NONE',  ( -957.2086549536782059, 47.65337959301152893, -124.6807709998040679 ) ) ;
#2457=CARTESIAN_POINT ( 'NONE',  ( -1030.931480980267906, 117.9615145441170654, -124.6807709998043521 ) ) ;
#2463=EDGE_CURVE ( 'NONE', #915, #1185, #9148, .T. ) ;
#2471=CARTESIAN_POINT ( 'NONE',  ( -828.8285638327243987, 78.67432280806596623, -144.4023295390031194 ) ) ;
#2478=CARTESIAN_POINT ( 'NONE',  ( -902.4158961391586899, 71.79205886009079052, -149.7857175106635736 ) ) ;
#2490=CARTESIAN_POINT ( 'NONE',  ( -976.2517683711890868, 35.25052392388818134, -126.6442663926290777 ) ) ;
#2493=CARTESIAN_POINT ( 'NONE',  ( -1061.884876827091830, 80.20192378191423188, -94.48732055948617869 ) ) ;
#2502=CARTESIAN_POINT ( 'NONE',  ( -822.6948441016551214, 83.54682639321367787, -154.1324994421172505 ) ) ;
#2503=CARTESIAN_POINT ( 'NONE',  ( -1031.956718292106189, 74.21439239895558160, -95.06748246948035330 ) ) ;
#2516=CARTESIAN_POINT ( 'NONE',  ( -1060.756016675587944, 112.8516620848305934, -122.7172756069790864 ) ) ;
#2523=CARTESIAN_POINT ( 'NONE',  ( -1045.864486809339724, 115.5688325305733741, -124.6807709998043663 ) ) ;
#2527=CARTESIAN_POINT ( 'NONE',  ( -1024.256845364727496, 79.46673622094714062, -154.2940595301284930 ) ) ;
#2528=CARTESIAN_POINT ( 'NONE',  ( -828.1715959468244819, 76.17590192436176721, -143.8160639703675940 ) ) ;
#2532=CARTESIAN_POINT ( 'NONE',  ( -952.6992609796615170, 94.45070821375009018, -154.2940595301278961 ) ) ;
#2538=CARTESIAN_POINT ( 'NONE',  ( -1032.260242496265846, 61.00429285198246987, -149.7857175106635452 ) ) ;
#2558=CARTESIAN_POINT ( 'NONE',  ( -974.9912860506733523, 88.33816101283738931, -95.06748246948018277 ) ) ;
#2564=CARTESIAN_POINT ( 'NONE',  ( -821.3240427761263618, 83.01413755802123262, -154.2176382493157121 ) ) ;
#2565=CARTESIAN_POINT ( 'NONE',  ( -953.5758047008322364, 72.53746257253780527, -96.78565065507940801 ) ) ;
#2574=CARTESIAN_POINT ( 'NONE',  ( -819.8516439069035187, 75.62621158465508131, -154.6795882100938400 ) ) ;
#2577=CARTESIAN_POINT ( 'NONE',  ( -795.0000000000020464, 111.6133447792289530, -118.7903414690682524 ) ) ;
#2588=CARTESIAN_POINT ( 'NONE',  ( -1065.000000000004320, 98.77454568802519930, -149.7857175106631189 ) ) ;
#2595=CARTESIAN_POINT ( 'NONE',  ( -818.8285638327243987, 78.67432280806558254, -94.73795703228648790 ) ) ;
#2600=CARTESIAN_POINT ( 'NONE',  ( -1024.256845364727496, 79.46673622094714062, -154.2940595301284930 ) ) ;
#2604=AXIS2_PLACEMENT_3D ( 'NONE', #10062, #6293, #1656 ) ;
#2616=CARTESIAN_POINT ( 'NONE',  ( -1015.517346982276649, 86.95624952299064603, -94.48732055948629238 ) ) ;
#2619=CARTESIAN_POINT ( 'NONE',  ( -825.4446906002115156, 83.41738352290740011, -144.6308861023095460 ) ) ;
#2625=CARTESIAN_POINT ( 'NONE',  ( -1032.113539130918525, 67.34854938887495734, -96.78565065507952170 ) ) ;
#2639=CARTESIAN_POINT ( 'NONE',  ( -1054.380968608931425, 114.0683136310379524, -124.6807709998043663 ) ) ;
#2652=CARTESIAN_POINT ( 'NONE',  ( -952.4132309232853686, 101.5728619241206161, -152.5758913445289409 ) ) ;
#2653=CARTESIAN_POINT ( 'NONE',  ( -828.8205192779003028, 78.34647195564971867, -144.3449412327541665 ) ) ;
#2659=CARTESIAN_POINT ( 'NONE',  ( -821.6815100408632588, 89.78153722040215712, -152.5758913445288840 ) ) ;
#2664=CARTESIAN_POINT ( 'NONE',  ( -1055.176328965298808, 98.13059730676609149, -149.7857175106632326 ) ) ;
#2665=CARTESIAN_POINT ( 'NONE',  ( -975.3893330992545998, 71.12659035875127245, -154.2940595301280950 ) ) ;
#2667=VECTOR ( 'NONE', #5683, 1000.000000000000000 ) ;
#2684=CARTESIAN_POINT ( 'NONE',  ( -1038.283672687642365, 64.16172732404288581, -96.78565065507946485 ) ) ;
#2686=CARTESIAN_POINT ( 'NONE',  ( -825.1286147475053667, 83.51336106040547236, -144.6235354408674141 ) ) ;
#2695=CARTESIAN_POINT ( 'NONE',  ( -1065.000000000002501, 60.65002596136933732, -103.3307627799636350 ) ) ;
#2697=DIRECTION ( 'NONE',  ( 4.236366511936864528E-16, -1.000000000000000000, -5.522905491341393153E-16 ) ) ;
#2699=CARTESIAN_POINT ( 'NONE',  ( -795.0000000000043201, 82.00000000000039790, -124.6807709998041105 ) ) ;
#2709=CARTESIAN_POINT ( 'NONE',  ( -974.3195816561840275, 116.7169707472884141, -107.9061927053320602 ) ) ;
#2718=CARTESIAN_POINT ( 'NONE',  ( -1010.922847972425529, 120.6260792194948550, -124.6807709998039542 ) ) ;
#2721=CARTESIAN_POINT ( 'NONE',  ( -1025.595388641371756, 103.7168792382127975, -149.7857175106636021 ) ) ;
#2724=CARTESIAN_POINT ( 'NONE',  ( -1031.632959140996718, 88.47632675500395294, -154.2940595301282087 ) ) ;
#2727=CARTESIAN_POINT ( 'NONE',  ( -828.8285638327245124, 78.67432280806571043, -264.6807709998050200 ) ) ;
#2731=CARTESIAN_POINT ( 'NONE',  ( -1061.276350651670782, 98.40484402385492047, -149.7857175106635452 ) ) ;
#2732=CARTESIAN_POINT ( 'NONE',  ( -955.9230626098308221, 78.80814421416198456, -154.2940595301282372 ) ) ;
#2739=CARTESIAN_POINT ( 'NONE',  ( -1065.000000000000909, 56.89504896194504369, -141.4553492942757771 ) ) ;
#2752=CARTESIAN_POINT ( 'NONE',  ( -956.4793285278434496, 64.87563161486531271, -99.57582448894522997 ) ) ;
#2757=CARTESIAN_POINT ( 'NONE',  ( -991.8293279264742068, 119.7328159579556086, -136.2353035311976726 ) ) ;
#2763=CARTESIAN_POINT ( 'NONE',  ( -1065.000000000009095, 65.22545431197600863, -99.57582448894517313 ) ) ;
#2777=CARTESIAN_POINT ( 'NONE',  ( -1031.197907781702725, 107.2697845108577894, -103.3307627799635640 ) ) ;
#2785=CARTESIAN_POINT ( 'NONE',  ( -1015.209561144950953, 93.46821065761417913, -154.2940595301282656 ) ) ;
#2794=CARTESIAN_POINT ( 'NONE',  ( -1037.656130532295037, 99.96792753513321372, -149.7857175106633747 ) ) ;
#2795=CARTESIAN_POINT ( 'NONE',  ( -1013.120138696094841, 73.26074010992857666, -152.5758913445291682 ) ) ;
#2804=DIRECTION ( 'NONE',  ( -1.000000000000000000, 1.262554838833776231E-16, 0.000000000000000000 ) ) ;
#2811=CARTESIAN_POINT ( 'NONE',  ( -1048.206790403141440, 45.99070412075073477, -107.9061927053325007 ) ) ;
#2814=CARTESIAN_POINT ( 'NONE',  ( -1057.805062346506702, 42.77845103615944566, -130.5712005305404944 ) ) ;
#2821=CARTESIAN_POINT ( 'NONE',  ( -1021.293373424897709, 59.24127555818995461, -107.9061927053327281 ) ) ;
#2836=CARTESIAN_POINT ( 'NONE',  ( -1021.913416468816195, 116.8879375517085890, -113.1262384684096673 ) ) ;
#2843=CARTESIAN_POINT ( 'NONE',  ( -991.5701548301636876, 122.8678427087060214, -124.6807709998040536 ) ) ;
#2847=CARTESIAN_POINT ( 'NONE',  ( -1031.632959140996718, 88.47632675500395294, -154.2940595301282087 ) ) ;
#2852=CARTESIAN_POINT ( 'NONE',  ( -1030.931480980266770, 117.9615145441171933, -126.6442663926290777 ) ) ;
#2858=CARTESIAN_POINT ( 'NONE',  ( -1061.884876827093876, 80.20192378191431715, -154.8742214401230797 ) ) ;
#2868=CARTESIAN_POINT ( 'NONE',  ( -825.1499223856457093, 73.84923531294217014, -106.4169293550704793 ) ) ;
#2876=CARTESIAN_POINT ( 'NONE',  ( -1013.392840968506675, 67.31954129910425877, -99.57582448894551419 ) ) ;
#2877=CARTESIAN_POINT ( 'NONE',  ( -828.8208027857029947, 78.99693817035523580, -104.9068376039975590 ) ) ;
#2879=CARTESIAN_POINT ( 'NONE',  ( -1021.607260580477828, 54.24386729702167997, -130.5712005305404659 ) ) ;
#2889=CARTESIAN_POINT ( 'NONE',  ( -902.0880155070191222, 62.23309906011806447, -107.9061927053322876 ) ) ;
#2898=CARTESIAN_POINT ( 'NONE',  ( -1011.418100375198719, 110.6663390795547599, -103.3307627799635782 ) ) ;
#2901=CARTESIAN_POINT ( 'NONE',  ( -823.1749794181308744, 110.1592441374104112, -141.4553492942763171 ) ) ;
#2904=CARTESIAN_POINT ( 'NONE',  ( -1037.337636019038882, 116.9882293220588991, -124.6807709998043521 ) ) ;
#2911=CARTESIAN_POINT ( 'NONE',  ( -1014.382386707152364, 110.5980896718283759, -146.0307792196445291 ) ) ;
#2916=CARTESIAN_POINT ( 'NONE',  ( -1013.901471336339000, 119.8325901201404804, -130.5712005305404944 ) ) ;
#2923=CARTESIAN_POINT ( 'NONE',  ( -822.5144771496200065, 73.83866123373456958, -106.4215885538521178 ) ) ;
#2924=CARTESIAN_POINT ( 'NONE',  ( -1021.046747802647246, 63.38047825189622841, -146.0307792196452681 ) ) ;
#2936=CARTESIAN_POINT ( 'NONE',  ( -1016.652307257391612, 63.31440937415304404, -103.3307627799640045 ) ) ;
#2937=CARTESIAN_POINT ( 'NONE',  ( -818.9856806503992175, 79.95950042232037447, -104.7825536331199743 ) ) ;
#2946=CARTESIAN_POINT ( 'NONE',  ( -956.4793285278434496, 64.87563161486531271, -99.57582448894522997 ) ) ;
#2947=CARTESIAN_POINT ( 'NONE',  ( -823.8285638327243987, 78.67432280806571043, -264.6807709998050200 ) ) ;
#2957=CARTESIAN_POINT ( 'NONE',  ( -1022.124201078493229, 113.7707856953083478, -107.9061927053324013 ) ) ;
#2960=CARTESIAN_POINT ( 'NONE',  ( -795.0000000000047748, 112.0000000000007532, -124.6807709998042384 ) ) ;
#2962=DIRECTION ( 'NONE',  ( 1.000000000000000000, -1.262554838833776231E-16, 0.000000000000000000 ) ) ;
#2965=CARTESIAN_POINT ( 'NONE',  ( -1014.170783943998003, 114.7803637426474808, -141.4553492942763171 ) ) ;
#2970=EDGE_CURVE ( 'NONE', #9730, #178, #9103, .T. ) ;
#2979=CARTESIAN_POINT ( 'NONE',  ( -819.0854767918264088, 77.05939038872190849, -105.2981374327915347 ) ) ;
#2980=CARTESIAN_POINT ( 'NONE',  ( -954.2862664537763067, 55.36536439393486830, -141.4553492942758908 ) ) ;
#2988=CARTESIAN_POINT ( 'NONE',  ( -817.2011019090375612, 28.13185037056175375, -130.5712005305403238 ) ) ;
#2993=CARTESIAN_POINT ( 'NONE',  ( -1013.120138696091999, 73.26074010992823560, -96.78565065507963538 ) ) ;
#2994=CARTESIAN_POINT ( 'NONE',  ( -828.7652305532269565, 79.48420453549685760, -104.8389787515932881 ) ) ;
#3005=CARTESIAN_POINT ( 'NONE',  ( -957.1839320239914741, 48.17551948191501765, -118.7903414690682951 ) ) ;
#3011=CARTESIAN_POINT ( 'NONE',  ( -904.0006525278403160, 119.6095687608906672, -107.9061927053323160 ) ) ;
#3018=CARTESIAN_POINT ( 'NONE',  ( -1046.457602311629898, 98.67849639484570901, -99.57582448894517313 ) ) ;
#3019=CARTESIAN_POINT ( 'NONE',  ( -1017.840614713428863, 119.3387310954208118, -130.5712005305402954 ) ) ;
#3021=CARTESIAN_POINT ( 'NONE',  ( -823.7697810748813936, 117.7733807739867871, -122.7172756069790438 ) ) ;
#3028=CARTESIAN_POINT ( 'NONE',  ( -1065.000000000003411, 103.3499740386315580, -146.0307792196444154 ) ) ;
#3037=CARTESIAN_POINT ( 'NONE',  ( -1062.301584968959560, 67.66927912025090563, -152.5758913445295377 ) ) ;
#3044=CARTESIAN_POINT ( 'NONE',  ( -1021.483947769362658, 56.15424078096121008, -136.2353035311990368 ) ) ;
#3051=CARTESIAN_POINT ( 'NONE',  ( -1062.923339974269538, 49.86928741160662071, -113.1262384684094968 ) ) ;
#3056=CARTESIAN_POINT ( 'NONE',  ( -826.4716404759357147, 74.42688921697002513, -154.6727229035019775 ) ) ;
#3062=CARTESIAN_POINT ( 'NONE',  ( -1032.658196452834773, 44.72920460984212809, -122.7172756069792143 ) ) ;
#3068=CARTESIAN_POINT ( 'NONE',  ( -1011.211222789223370, 114.9684118750912489, -107.9061927053323870 ) ) ;
#3074=CARTESIAN_POINT ( 'NONE',  ( -1022.719357623492556, 104.5170332807322922, -99.57582448894488891 ) ) ;
#3085=CARTESIAN_POINT ( 'NONE',  ( -1021.913416468810851, 116.8879375517085464, -136.2353035311978431 ) ) ;
#3093=CARTESIAN_POINT ( 'NONE',  ( -1024.691966601152672, 118.8493250655916142, -124.6807709998039400 ) ) ;
#3095=CARTESIAN_POINT ( 'NONE',  ( -795.0000000000046612, 103.3499740386315864, -146.0307792196441312 ) ) ;
#3101=CARTESIAN_POINT ( 'NONE',  ( -1032.391769651406321, 55.42093464310143247, -146.0307792196449839 ) ) ;
#3107=DIRECTION ( 'NONE',  ( 0.000000000000000000, 5.522905491341382306E-16, 1.000000000000000000 ) ) ;
#3108=CARTESIAN_POINT ( 'NONE',  ( -976.1667687410197232, 38.51511931707989334, -113.1262384684093263 ) ) ;
#3112=CARTESIAN_POINT ( 'NONE',  ( -823.5011105148523711, 73.67440276501611152, -154.6460142633133614 ) ) ;
#3116=CARTESIAN_POINT ( 'NONE',  ( -954.5692209181586350, 49.02792041507773746, -122.7172756069790580 ) ) ;
#3123=CARTESIAN_POINT ( 'NONE',  ( -1025.296800000965050, 108.9225844456047696, -103.3307627799635782 ) ) ;
#3127=ORIENTED_EDGE ( 'NONE', *, *, #4480, .T. ) ;
#3129=CARTESIAN_POINT ( 'NONE',  ( -993.0619804577127070, 103.7129695969639442, -99.57582448894480365 ) ) ;
#3132=CARTESIAN_POINT ( 'NONE',  ( -1065.000000000005912, 111.6133447792291093, -130.5712005305407217 ) ) ;
#3133=CARTESIAN_POINT ( 'NONE',  ( -1031.000617048993718, 115.3267894020686697, -136.2353035311981557 ) ) ;
#3137=CARTESIAN_POINT ( 'NONE',  ( -1037.348432443215870, 116.4729352038311987, -118.7903414690680961 ) ) ;
#3148=CARTESIAN_POINT ( 'NONE',  ( -823.7697810748812799, 117.7733807739867871, -124.6807709998041531 ) ) ;
#3150=CARTESIAN_POINT ( 'NONE',  ( -974.3195816561885749, 116.7169707472886842, -141.4553492942758055 ) ) ;
#3158=CARTESIAN_POINT ( 'NONE',  ( -1048.040919118598822, 50.77060569800413248, -146.0307792196448986 ) ) ;
#3162=CARTESIAN_POINT ( 'NONE',  ( -828.7970580965601357, 78.02475450683051861, -94.74435982432032688 ) ) ;
#3164=CARTESIAN_POINT ( 'NONE',  ( -1025.806732200655688, 55.05754055295027172, -136.2353035311988663 ) ) ;
#3166=CARTESIAN_POINT ( 'NONE',  ( -1021.637154595298057, 53.81063926482157456, -122.7172756069792285 ) ) ;
#3168=CARTESIAN_POINT ( 'NONE',  ( -976.1667687410277949, 38.51511931708004965, -136.2353035311986957 ) ) ;
#3176=CARTESIAN_POINT ( 'NONE',  ( -1057.832023714520119, 42.29985473022490794, -126.6442663926294330 ) ) ;
#3179=CARTESIAN_POINT ( 'NONE',  ( -926.9570750291553622, 111.1083136274928620, -99.57582448894491733 ) ) ;
#3185=CARTESIAN_POINT ( 'NONE',  ( -994.1998135634719347, 88.30642396300639518, -95.06748246948001224 ) ) ;
#3187=CARTESIAN_POINT ( 'NONE',  ( -1024.722591077094876, 118.3980260646368379, -130.5712005305404944 ) ) ;
#3188=CARTESIAN_POINT ( 'NONE',  ( -1013.875822516558969, 120.2710389253236940, -126.6442663926291061 ) ) ;
#3193=CARTESIAN_POINT ( 'NONE',  ( -1045.967528061859412, 112.8272211019270230, -113.1262384684098663 ) ) ;
#3194=CARTESIAN_POINT ( 'NONE',  ( -828.8285638327240576, 78.67432280806576728, -94.77914401073080342 ) ) ;
#3196=CARTESIAN_POINT ( 'NONE',  ( -928.4368846968633306, 59.55532739646334051, -124.6807709998041105 ) ) ;
#3199=EDGE_LOOP ( 'NONE', ( #3778, #1566 ) ) ;
#3201=DIRECTION ( 'NONE',  ( 1.000000000000000000, 4.236366511936864528E-16, 3.037002292462560327E-31 ) ) ;
#3205=CARTESIAN_POINT ( 'NONE',  ( -951.9057582426059980, 113.9552214607316216, -146.0307792196438754 ) ) ;
#3209=CARTESIAN_POINT ( 'NONE',  ( -995.4135022096103285, 71.70161378084171133, -154.2940595301282656 ) ) ;
#3213=CARTESIAN_POINT ( 'NONE',  ( -823.1773471095956438, 73.70622229620707344, -94.71566886200753288 ) ) ;
#3219=CARTESIAN_POINT ( 'NONE',  ( -1038.506348936321501, 51.71309463382193883, -146.0307792196451260 ) ) ;
#3223=CARTESIAN_POINT ( 'NONE',  ( -1057.693846703447207, 44.87596864925360052, -113.1262384684097100 ) ) ;
#3224=CARTESIAN_POINT ( 'NONE',  ( -828.8285638327240576, 78.67432280806576728, -94.77914401073080342 ) ) ;
#3230=CARTESIAN_POINT ( 'NONE',  ( -1014.107508992752514, 52.59077491224128664, -118.7903414690682951 ) ) ;
#3236=CARTESIAN_POINT ( 'NONE',  ( -1014.632462699974781, 105.5176738732103132, -99.57582448894522997 ) ) ;
#3242=CARTESIAN_POINT ( 'NONE',  ( -974.6181169426257611, 104.3135445892214506, -99.57582448894483207 ) ) ;
#3244=CARTESIAN_POINT ( 'NONE',  ( -954.0688428831344936, 124.4732772249357282, -130.5712005305405796 ) ) ;
#3245=CARTESIAN_POINT ( 'NONE',  ( -823.7697810748812799, 117.7733807739867871, -124.6807709998041531 ) ) ;
#3269=ORIENTED_EDGE ( 'NONE', *, *, #5649, .T. ) ;
#3277=CARTESIAN_POINT ( 'NONE',  ( -1065.000000000001364, 65.22545431197576704, -149.7857175106635168 ) ) ;
#3283=CARTESIAN_POINT ( 'NONE',  ( -1017.027421246622112, 56.01181809833683900, -113.1262384684095537 ) ) ;
#3286=CARTESIAN_POINT ( 'NONE',  ( -828.8285638327250808, 79.00071959000507604, -94.79793468034198156 ) ) ;
#3296=CARTESIAN_POINT ( 'NONE',  ( -821.6815100408621220, 89.78153722040228502, -96.78565065507908116 ) ) ;
#3314=CARTESIAN_POINT ( 'NONE',  ( -819.4886053768613010, 81.17856470051358997, -94.91880207566623540 ) ) ;
#3316=ORIENTED_EDGE ( 'NONE', *, *, #5104, .F. ) ;
#3318=CARTESIAN_POINT ( 'NONE',  ( -823.7697810748826441, 117.7733807739869292, -126.6442663926291914 ) ) ;
#3328=CARTESIAN_POINT ( 'NONE',  ( -1031.956718292102323, 74.21439239895576634, -154.2940595301282656 ) ) ;
#3329=CARTESIAN_POINT ( 'NONE',  ( -825.4626643026906549, 73.93730723265454685, -142.9841191000405729 ) ) ;
#3339=CARTESIAN_POINT ( 'NONE',  ( -975.7625022073049195, 55.15120678236734619, -149.7857175106636589 ) ) ;
#3351=CARTESIAN_POINT ( 'NONE',  ( -1022.719357623492556, 104.5170332807322922, -99.57582448894488891 ) ) ;
#3360=CARTESIAN_POINT ( 'NONE',  ( -828.8285638327247398, 79.00071603608273563, -154.5636075238658691 ) ) ;
#3361=CARTESIAN_POINT ( 'NONE',  ( -975.3893330992572146, 71.12659035875115876, -95.06748246948035330 ) ) ;
#3366=CARTESIAN_POINT ( 'NONE',  ( -818.8285638327240576, 78.67432280806558254, -104.9592124606052295 ) ) ;
#3372=CARTESIAN_POINT ( 'NONE',  ( -852.8175266017512968, 121.6828083272127685, -122.7172756069790438 ) ) ;
#3381=CARTESIAN_POINT ( 'NONE',  ( -1015.825132819589953, 80.44428838836770979, -154.2940595301284645 ) ) ;
#3390=CARTESIAN_POINT ( 'NONE',  ( -795.0000000000071623, 60.65002596136950075, -146.0307792196447565 ) ) ;
#3406=CARTESIAN_POINT ( 'NONE',  ( -1047.392513188126713, 70.23666496464434772, -95.06748246948035330 ) ) ;
#3410=CARTESIAN_POINT ( 'NONE',  ( -795.0000000000048885, 52.00000000000024158, -124.6807709998040821 ) ) ;
#3419=CARTESIAN_POINT ( 'NONE',  ( -825.1280624195762812, 83.51352241364627105, -154.1197328629658045 ) ) ;
#3420=CARTESIAN_POINT ( 'NONE',  ( -1047.392513188126713, 70.23666496464434772, -95.06748246948035330 ) ) ;
#3424=CARTESIAN_POINT ( 'NONE',  ( -951.4198147059590838, 125.0824040815807194, -126.6442663926291345 ) ) ;
#3432=CARTESIAN_POINT ( 'NONE',  ( -976.2517683711889731, 35.25052392388816713, -124.6807709998040394 ) ) ;
#3433=CARTESIAN_POINT ( 'NONE',  ( -818.9957115137622168, 77.38185006597193194, -154.6675616934836057 ) ) ;
#3436=CARTESIAN_POINT ( 'NONE',  ( -974.1288507787422759, 124.2142274477005657, -124.6807709998040110 ) ) ;
#3438=EDGE_CURVE ( 'NONE', #178, #5809, #2164, .T. ) ;
#3446=ORIENTED_EDGE ( 'NONE', *, *, #2102, .F. ) ;
#3455=CARTESIAN_POINT ( 'NONE',  ( -818.8285638327245124, 78.34431818532443970, -94.72265437454855430 ) ) ;
#3457=CARTESIAN_POINT ( 'NONE',  ( -795.0000000000011369, 65.22545431197602284, -149.7857175106635452 ) ) ;
#3474=CARTESIAN_POINT ( 'NONE',  ( -1012.828629370415570, 79.69572830938430741, -95.06748246948046699 ) ) ;
#3477=ORIENTED_EDGE ( 'NONE', *, *, #9611, .F. ) ;
#3479=EDGE_CURVE ( 'NONE', #5145, #8436, #902, .T. ) ;
#3483=CARTESIAN_POINT ( 'NONE',  ( -828.5731522051593174, 80.28512761734042158, -154.4691854747994171 ) ) ;
#3484=CARTESIAN_POINT ( 'NONE',  ( -1020.082665824770629, 80.34198733739781062, -95.06748246948050962 ) ) ;
#3497=CARTESIAN_POINT ( 'NONE',  ( -1054.407929976941432, 113.5897173251036207, -118.7903414690678261 ) ) ;
#3507=CARTESIAN_POINT ( 'NONE',  ( -1025.928429817215147, 97.79385104913471594, -152.5758913445291398 ) ) ;
#3508=CARTESIAN_POINT ( 'NONE',  ( -827.8145948178575964, 75.63860347950591745, -143.6442145102269592 ) ) ;
#3519=CARTESIAN_POINT ( 'NONE',  ( -1038.283672687649414, 64.16172732404312740, -152.5758913445294240 ) ) ;
#3529=DIRECTION ( 'NONE',  ( 0.000000000000000000, 1.000000000000000000, 6.938893903907169213E-16 ) ) ;
#3533=CARTESIAN_POINT ( 'NONE',  ( -902.8257469293350823, 84.21185948885704420, -95.06748246948052383 ) ) ;
#3555=CARTESIAN_POINT ( 'NONE',  ( -991.6207251904191935, 122.2801902404845151, -118.7903414690677124 ) ) ;
#3566=CARTESIAN_POINT ( 'NONE',  ( -820.4595805503685142, 72.64106675864371709, -154.8742214401225397 ) ) ;
#3570=CARTESIAN_POINT ( 'NONE',  ( -903.4746773471192682, 104.0883302344920480, -152.5758913445288272 ) ) ;
#3576=CARTESIAN_POINT ( 'NONE',  ( -1027.375436305353333, 71.63039521860234515, -152.5758913445296230 ) ) ;
#3579=CIRCLE ( 'NONE', #4600, 30.00000000000021316 ) ;
#3598=CARTESIAN_POINT ( 'NONE',  ( -1062.301584968951602, 67.66927912025059300, -96.78565065507969223 ) ) ;
#3607=CARTESIAN_POINT ( 'NONE',  ( -997.0443963278638648, 49.75991663364290929, -103.3307627799637487 ) ) ;
#3623=CARTESIAN_POINT ( 'NONE',  ( -1013.875822516560447, 120.2710389253235519, -124.6807709998039257 ) ) ;
#3633=CARTESIAN_POINT ( 'NONE',  ( -1030.931480980267906, 117.9615145441170654, -124.6807709998043521 ) ) ;
#3636=CARTESIAN_POINT ( 'NONE',  ( -1065.000000000007731, 93.55451860843886891, -152.5758913445290830 ) ) ;
#3641=CARTESIAN_POINT ( 'NONE',  ( -903.2629211055218548, 97.63080833215174437, -154.2940595301276971 ) ) ;
#3644=CARTESIAN_POINT ( 'NONE',  ( -819.0860990673882043, 77.05720446847304572, -94.68731928646728591 ) ) ;
#3648=CARTESIAN_POINT ( 'NONE',  ( -1065.000000000008868, 82.00000000000028422, -154.8742214401231081 ) ) ;
#3656=CARTESIAN_POINT ( 'NONE',  ( -827.1569714199418968, 74.92915896789017438, -105.9707980921570112 ) ) ;
#3657=CARTESIAN_POINT ( 'NONE',  ( -928.3598895238005753, 61.90886769853032945, -136.2353035311983263 ) ) ;
#3671=CARTESIAN_POINT ( 'NONE',  ( -1025.595947590972401, 58.17469240935120922, -107.9061927053327707 ) ) ;
#3680=CARTESIAN_POINT ( 'NONE',  ( -956.7203770923135835, 58.97922774997691420, -103.3307627799636919 ) ) ;
#3696=CARTESIAN_POINT ( 'NONE',  ( -852.9318753287178652, 113.3383058689773151, -107.9061927053323302 ) ) ;
#3705=CARTESIAN_POINT ( 'NONE',  ( -795.0000000000094360, 82.00000000000081002, -154.8742214401225397 ) ) ;
#3708=CARTESIAN_POINT ( 'NONE',  ( -1025.928429817215147, 97.79385104913471594, -152.5758913445291398 ) ) ;
#3715=CARTESIAN_POINT ( 'NONE',  ( -1031.956718292102323, 74.21439239895576634, -154.2940595301282656 ) ) ;
#3717=CIRCLE ( 'NONE', #6283, 30.00000000000021316 ) ;
#3719=VECTOR ( 'NONE', #6238, 1000.000000000000000 ) ;
#3721=CARTESIAN_POINT ( 'NONE',  ( -827.1410867119041086, 82.43389265416672629, -144.6774099844745365 ) ) ;
#3725=CARTESIAN_POINT ( 'NONE',  ( -901.9718911164696920, 59.00785292138922244, -136.2353035311984115 ) ) ;
#3735=CARTESIAN_POINT ( 'NONE',  ( -1062.810894920125520, 52.92335929224832825, -107.9061927053327139 ) ) ;
#3738=CARTESIAN_POINT ( 'NONE',  ( -817.1493800258450619, 27.50875274330017461, -126.6442663926291630 ) ) ;
#3739=CARTESIAN_POINT ( 'NONE',  ( -821.6112282492948680, 83.16771792585157641, -144.6470480974983843 ) ) ;
#3746=CARTESIAN_POINT ( 'NONE',  ( -1047.844889418690855, 56.55730854968127375, -99.57582448894520155 ) ) ;
#3757=CARTESIAN_POINT ( 'NONE',  ( -1025.044148074454370, 113.2108726315405960, -107.9061927053325007 ) ) ;
#3762=CARTESIAN_POINT ( 'NONE',  ( -1010.922847972425529, 120.6260792194948550, -124.6807709998039542 ) ) ;
#3768=CARTESIAN_POINT ( 'NONE',  ( -927.4753839990684128, 92.66010094724849466, -154.8742214401223691 ) ) ;
#3775=CARTESIAN_POINT ( 'NONE',  ( -1012.828629370413182, 79.69572830938452057, -154.2940595301284361 ) ) ;
#3778=ORIENTED_EDGE ( 'NONE', *, *, #2102, .T. ) ;
#3779=CARTESIAN_POINT ( 'NONE',  ( -825.6238610960883761, 74.00482032089516338, -106.3482309385110511 ) ) ;
#3785=CARTESIAN_POINT ( 'NONE',  ( -1065.000000000006366, 82.00000000000036948, -124.6807709998044231 ) ) ;
#3792=CARTESIAN_POINT ( 'NONE',  ( -953.8433812051914629, 65.95343150956773570, -99.57582448894520155 ) ) ;
#3793=CARTESIAN_POINT ( 'NONE',  ( -827.1368241426298482, 82.43785830827036420, -104.6842000310834777 ) ) ;
#3795=CARTESIAN_POINT ( 'NONE',  ( -1057.832023714520119, 42.29985473022490794, -126.6442663926294330 ) ) ;
#3802=CARTESIAN_POINT ( 'NONE',  ( -954.2862664537825594, 55.36536439393501041, -107.9061927053324439 ) ) ;
#3816=CARTESIAN_POINT ( 'NONE',  ( -926.6866529578969676, 120.3119365386820192, -107.9061927053322734 ) ) ;
#3818=CARTESIAN_POINT ( 'NONE',  ( -1030.944970944897250, 117.4714819019839354, -130.5712005305406649 ) ) ;
#3823=CARTESIAN_POINT ( 'NONE',  ( -1054.380968608931425, 114.0683136310379524, -124.6807709998043663 ) ) ;
#3827=CARTESIAN_POINT ( 'NONE',  ( -1061.104375862961888, 103.3839434440459968, -146.0307792196447565 ) ) ;
#3846=CARTESIAN_POINT ( 'NONE',  ( -902.2382941300837729, 66.55116351576596401, -146.0307792196448986 ) ) ;
#3853=AXIS2_PLACEMENT_3D ( 'NONE', #8253, #6326, #1823 ) ;
#3857=CARTESIAN_POINT ( 'NONE',  ( -1048.040919118596321, 50.77060569800394063, -103.3307627799636919 ) ) ;
#3858=PLANE ( 'NONE',  #10505 ) ;
#3859=CARTESIAN_POINT ( 'NONE',  ( -1021.637154595298057, 53.81063926482157456, -126.6442663926291630 ) ) ;
#3862=CARTESIAN_POINT ( 'NONE',  ( -826.3405481598731512, 83.00984762678820061, -144.6560901833814796 ) ) ;
#3868=CARTESIAN_POINT ( 'NONE',  ( -975.7625022073081027, 55.15120678236761620, -99.57582448894500260 ) ) ;
#3872=CARTESIAN_POINT ( 'NONE',  ( -795.0000000000065938, 109.8950841424301217, -113.1262384684096105 ) ) ;
#3880=CARTESIAN_POINT ( 'NONE',  ( -1046.095701327177267, 109.2451008237761982, -107.9061927053324439 ) ) ;
#3883=CARTESIAN_POINT ( 'NONE',  ( -974.2138504089066373, 120.9496320545085695, -136.2353035311977010 ) ) ;
#3891=CARTESIAN_POINT ( 'NONE',  ( -1065.000000000003411, 103.3499740386315580, -146.0307792196444154 ) ) ;
#3896=CARTESIAN_POINT ( 'NONE',  ( -1031.086615573508880, 111.8776252365151009, -141.4553492942759760 ) ) ;
#3905=CARTESIAN_POINT ( 'NONE',  ( -928.1401715909056520, 69.16346707077036626, -146.0307792196452965 ) ) ;
#3914=CARTESIAN_POINT ( 'NONE',  ( -957.0819499390250940, 50.45265437475578807, -136.2353035311988663 ) ) ;
#3920=CARTESIAN_POINT ( 'NONE',  ( -819.2376510598700179, 55.50059629688461627, -96.78565065507937959 ) ) ;
#3921=CARTESIAN_POINT ( 'NONE',  ( -826.8820017809032379, 82.64709913614477443, -104.6904163631604092 ) ) ;
#3926=CARTESIAN_POINT ( 'NONE',  ( -820.7761598878998939, 74.70052632655239222, -154.6666544911500694 ) ) ;
#3931=CARTESIAN_POINT ( 'NONE',  ( -954.5446161821273563, 49.54000128949434867, -118.7903414690681103 ) ) ;
#3936=CARTESIAN_POINT ( 'NONE',  ( -904.1167769183953169, 122.8348148996191611, -113.1262384684093263 ) ) ;
#3939=CARTESIAN_POINT ( 'NONE',  ( -818.8285638327242850, 78.67432280806571043, -264.6807709998050200 ) ) ;
#3941=CARTESIAN_POINT ( 'NONE',  ( -1019.365209469143679, 93.24061105504411273, -95.06748246948018277 ) ) ;
#3943=CARTESIAN_POINT ( 'NONE',  ( -1011.051362836436624, 118.1813008219153716, -136.2353035311982126 ) ) ;
#3951=CARTESIAN_POINT ( 'NONE',  ( -1065.000000000002501, 109.8950841424301359, -136.2353035311980136 ) ) ;
#3957=CARTESIAN_POINT ( 'NONE',  ( -1014.632462699976486, 105.5176738732105690, -149.7857175106636589 ) ) ;
#3965=CARTESIAN_POINT ( 'NONE',  ( -902.4158961391586899, 71.79205886009079052, -149.7857175106635736 ) ) ;
#3977=LINE ( 'NONE', #11585, #929 ) ;
#3979=CARTESIAN_POINT ( 'NONE',  ( -928.2641150402301946, 65.00826535581501275, -107.9061927053325576 ) ) ;
#3980=CARTESIAN_POINT ( 'NONE',  ( -826.0484035456470338, 83.16661265238063550, -104.7144245788475558 ) ) ;
#3986=CARTESIAN_POINT ( 'NONE',  ( -828.3859444281002880, 76.61103737358284604, -154.6660282174712222 ) ) ;
#3989=PRODUCT_CONTEXT ( 'NONE', #11196, 'mechanical' ) ;
#3992=CARTESIAN_POINT ( 'NONE',  ( -1025.806732200646138, 55.05754055295012961, -113.1262384684095537 ) ) ;
#3996=CARTESIAN_POINT ( 'NONE',  ( -1022.124201078493229, 113.7707856953083478, -107.9061927053324013 ) ) ;
#4003=CARTESIAN_POINT ( 'NONE',  ( -952.1456544189251190, 108.1568929870907141, -99.57582448894486049 ) ) ;
#4006=CARTESIAN_POINT ( 'NONE',  ( -1060.773655115453948, 112.4236047030759238, -130.5712005305406080 ) ) ;
#4010=CARTESIAN_POINT ( 'NONE',  ( -1021.743962174751232, 119.2557508373789403, -122.7172756069789585 ) ) ;
#4016=CARTESIAN_POINT ( 'NONE',  ( -926.6866529579010603, 120.3119365386823034, -141.4553492942759760 ) ) ;
#4020=CARTESIAN_POINT ( 'NONE',  ( -991.5701548301635739, 122.8678427087061493, -126.6442663926292056 ) ) ;
#4022=CARTESIAN_POINT ( 'NONE',  ( -1025.044148074459827, 113.2108726315406813, -141.4553492942762318 ) ) ;
#4030=CARTESIAN_POINT ( 'NONE',  ( -956.9243412622475944, 54.10650223846812423, -141.4553492942761181 ) ) ;
#4040=CARTESIAN_POINT ( 'NONE',  ( -1038.664246639927342, 43.28664065472985811, -136.2353035311990084 ) ) ;
#4047=CARTESIAN_POINT ( 'NONE',  ( -901.9718911164643487, 59.00785292138902349, -113.1262384684096105 ) ) ;
#4054=SHAPE_DEFINITION_REPRESENTATION ( #6054, #6213 ) ;
#4057=CARTESIAN_POINT ( 'NONE',  ( -1057.832023714519210, 42.29985473022490794, -122.7172756069794559 ) ) ;
#4063=CARTESIAN_POINT ( 'NONE',  ( -1014.382386707157252, 110.5980896718282196, -103.3307627799636350 ) ) ;
#4067=DIRECTION ( 'NONE',  ( 0.000000000000000000, 1.000000000000000000, 6.938893903907169213E-16 ) ) ;
#4069=CARTESIAN_POINT ( 'NONE',  ( -1011.662592067698938, 105.4443429699071828, -99.57582448894505944 ) ) ;
#4070=EDGE_CURVE ( 'NONE', #5809, #140, #7211, .T. ) ;
#4072=CARTESIAN_POINT ( 'NONE',  ( -991.6207251904210125, 122.2801902404846714, -130.5712005305406080 ) ) ;
#4075=CARTESIAN_POINT ( 'NONE',  ( -991.6207251904191935, 122.2801902404845151, -118.7903414690677124 ) ) ;
#4088=CARTESIAN_POINT ( 'NONE',  ( -1018.154501869017849, 114.3413228342528214, -141.4553492942762887 ) ) ;
#4095=CARTESIAN_POINT ( 'NONE',  ( -818.6751755801125228, 47.70925804672287995, -149.7857175106634884 ) ) ;
#4099=CARTESIAN_POINT ( 'NONE',  ( -825.1267440042464614, 73.83480927677597094, -94.70504551274875382 ) ) ;
#4101=CARTESIAN_POINT ( 'NONE',  ( -1048.334963668468163, 42.40858384259928471, -136.2353035311987242 ) ) ;
#4105=CARTESIAN_POINT ( 'NONE',  ( -954.4431216459856842, 51.77564274757639140, -113.1262384684095537 ) ) ;
#4109=CARTESIAN_POINT ( 'NONE',  ( -828.3857845960920940, 80.73794319005740761, -94.93252152554778434 ) ) ;
#4112=CARTESIAN_POINT ( 'NONE',  ( -827.1306228376723766, 74.90530319234137835, -154.6796240013121064 ) ) ;
#4116=CARTESIAN_POINT ( 'NONE',  ( -1057.805062346511704, 42.77845103615958067, -118.7903414690684087 ) ) ;
#4121=CARTESIAN_POINT ( 'NONE',  ( -926.8105964072291272, 116.1567348237266515, -103.3307627799635213 ) ) ;
#4126=CARTESIAN_POINT ( 'NONE',  ( -1031.476138302181198, 95.34216976508436403, -96.78565065507929432 ) ) ;
#4128=CARTESIAN_POINT ( 'NONE',  ( -1013.875822516560447, 120.2710389253235519, -124.6807709998039257 ) ) ;
#4138=CARTESIAN_POINT ( 'NONE',  ( -1017.158871447982392, 53.64146012065780411, -124.6807709998041389 ) ) ;
#4144=CARTESIAN_POINT ( 'NONE',  ( -955.0000000000038654, 82.00000000000036948, -124.6807709998041673 ) ) ;
#4145=CARTESIAN_POINT ( 'NONE',  ( -1021.743962174751232, 119.2557508373790824, -126.6442663926290209 ) ) ;
#4157=CARTESIAN_POINT ( 'NONE',  ( -818.1708872189602744, 40.82851623284160070, -146.0307792196448702 ) ) ;
#4159=ORIENTED_EDGE ( 'NONE', *, *, #8755, .T. ) ;
#4162=CARTESIAN_POINT ( 'NONE',  ( -1032.644706488208840, 45.21923725197571997, -118.7903414690683519 ) ) ;
#4164=CARTESIAN_POINT ( 'NONE',  ( -825.1270161104789622, 83.51388719778367431, -95.24185468551783629 ) ) ;
#4166=CARTESIAN_POINT ( 'NONE',  ( -828.8285638327247398, 78.67432280806576728, -154.5823979888776591 ) ) ;
#4170=CARTESIAN_POINT ( 'NONE',  ( -1021.483947769352199, 56.15424078096101113, -113.1262384684096105 ) ) ;
#4172=CARTESIAN_POINT ( 'NONE',  ( -1023.078931369429029, 98.73915068298381925, -96.78565065507928011 ) ) ;
#4179=ORIENTED_EDGE ( 'NONE', *, *, #5104, .T. ) ;
#4180=CARTESIAN_POINT ( 'NONE',  ( -974.7984820115178763, 96.63273410478059589, -96.78565065507896747 ) ) ;
#4183=CARTESIAN_POINT ( 'NONE',  ( -1054.380968608929606, 114.0683136310380803, -126.6442663926291345 ) ) ;
#4188=CARTESIAN_POINT ( 'NONE',  ( -1054.519145619997744, 111.4921997120089401, -113.1262384684101079 ) ) ;
#4192=CARTESIAN_POINT ( 'NONE',  ( -1032.658196452834090, 44.72920460984212809, -124.6807709998042100 ) ) ;
#4194=CARTESIAN_POINT ( 'NONE',  ( -818.8285638327246261, 79.00509885246378872, -94.75329546164918781 ) ) ;
#4199=CARTESIAN_POINT ( 'NONE',  ( -1021.743962174751232, 119.2557508373789403, -124.6807709998040110 ) ) ;
#4212=CARTESIAN_POINT ( 'NONE',  ( -820.5263375362879970, 74.90579914177446597, -94.69102061099690104 ) ) ;
#4215=CARTESIAN_POINT ( 'NONE',  ( -1025.000791045970800, 67.42844482392692385, -149.7857175106636305 ) ) ;
#4220=CARTESIAN_POINT ( 'NONE',  ( -928.4218612484631876, 59.99049470396640515, -118.7903414690680535 ) ) ;
#4222=CARTESIAN_POINT ( 'NONE',  ( -825.4392429272181744, 83.41914585070148291, -95.23026386004784172 ) ) ;
#4227=CARTESIAN_POINT ( 'NONE',  ( -795.0000000000036380, 52.00000000000027711, -126.6442663926292624 ) ) ;
#4236=CARTESIAN_POINT ( 'NONE',  ( -927.1204550305436669, 105.3607176047075029, -96.78565065507918064 ) ) ;
#4249=CARTESIAN_POINT ( 'NONE',  ( -996.0013826475885708, 63.70094029248571132, -96.78565065507963538 ) ) ;
#4283=CARTESIAN_POINT ( 'NONE',  ( -1013.392840968502924, 67.31954129910421614, -149.7857175106636873 ) ) ;
#4291=CARTESIAN_POINT ( 'NONE',  ( -826.4736066356965694, 82.92053275976070381, -95.16834756612315971 ) ) ;
#4299=CARTESIAN_POINT ( 'NONE',  ( -1061.104375862967800, 103.3839434440458547, -103.3307627799635924 ) ) ;
#4308=CARTESIAN_POINT ( 'NONE',  ( -828.8285638327247398, 78.67432280806576728, -154.5823979888776591 ) ) ;
#4309=CARTESIAN_POINT ( 'NONE',  ( -1012.527716518103489, 86.38194213450553605, -94.48732055948642028 ) ) ;
#4311=CARTESIAN_POINT ( 'NONE',  ( -1024.691966601152672, 118.8493250655916142, -124.6807709998039400 ) ) ;
#4317=CARTESIAN_POINT ( 'NONE',  ( -823.1736050761592196, 83.64219470983154281, -95.24653602621386028 ) ) ;
#4320=CARTESIAN_POINT ( 'NONE',  ( -823.7180591916842332, 117.1502831467252150, -118.7903414690680535 ) ) ;
#4332=CARTESIAN_POINT ( 'NONE',  ( -927.6556653798983234, 86.18751778479050074, -154.2940595301282656 ) ) ;
#4333=CARTESIAN_POINT ( 'NONE',  ( -828.8285638327246261, 78.51036871773322900, -144.3746817049001834 ) ) ;
#4337=CARTESIAN_POINT ( 'NONE',  ( -819.3359138399641779, 76.45573320715882915, -94.68090302126685742 ) ) ;
#4341=CARTESIAN_POINT ( 'NONE',  ( -1021.046747802647246, 63.38047825189622841, -146.0307792196452681 ) ) ;
#4358=CARTESIAN_POINT ( 'NONE',  ( -927.4753839990671622, 92.66010094724835255, -94.48732055948569553 ) ) ;
#4366=CARTESIAN_POINT ( 'NONE',  ( -826.0516380081095349, 83.16490949901579199, -154.1628641512737943 ) ) ;
#4367=CARTESIAN_POINT ( 'NONE',  ( -1027.019426772557381, 78.04595964998433999, -95.06748246948046699 ) ) ;
#4377=DIRECTION ( 'NONE',  ( 0.000000000000000000, 5.522905491341382306E-16, 1.000000000000000000 ) ) ;
#4378=CARTESIAN_POINT ( 'NONE',  ( -974.1288507787421622, 124.2142274477005657, -122.7172756069789017 ) ) ;
#4389=CARTESIAN_POINT ( 'NONE',  ( -1038.028607166442953, 78.75533988487831039, -154.8742214401230797 ) ) ;
#4390=CARTESIAN_POINT ( 'NONE',  ( -827.1548796934596339, 74.92718183615757255, -143.3900093790826418 ) ) ;
#4397=CARTESIAN_POINT ( 'NONE',  ( -1047.844889418685170, 56.55730854968103927, -149.7857175106634315 ) ) ;
#4407=EDGE_LOOP ( 'NONE', ( #1384, #4159, #415, #2025 ) ) ;
#4418=CARTESIAN_POINT ( 'NONE',  ( -1024.256845364730452, 79.46673622094698430, -95.06748246948041015 ) ) ;
#4424=ADVANCED_FACE ( 'NONE', ( #1711, #1643 ), #718, .F. ) ;
#4429=CARTESIAN_POINT ( 'NONE',  ( -824.4878712493014064, 83.64140073480777460, -154.1055574741608325 ) ) ;
#4430=CARTESIAN_POINT ( 'NONE',  ( -1024.641217300039216, 73.20632742167531148, -96.78565065507991960 ) ) ;
#4440=CARTESIAN_POINT ( 'NONE',  ( -823.5047064235034213, 114.4566975831562274, -136.2353035311979284 ) ) ;
#4443=CARTESIAN_POINT ( 'NONE',  ( -904.1919162299243453, 124.8346192645297918, -118.7903414690678119 ) ) ;
#4454=CARTESIAN_POINT ( 'NONE',  ( -1037.899050076299318, 86.18944477603574228, -154.2940595301282656 ) ) ;
#4457=CARTESIAN_POINT ( 'NONE',  ( -1011.935294340112478, 99.50314415908300703, -152.5758913445291967 ) ) ;
#4460=CARTESIAN_POINT ( 'NONE',  ( -818.8609195637731091, 78.01770880634862237, -94.71076406233586908 ) ) ;
#4465=CARTESIAN_POINT ( 'NONE',  ( -1062.301584968959560, 67.66927912025090563, -152.5758913445295377 ) ) ;
#4477=CARTESIAN_POINT ( 'NONE',  ( -1038.708781889657075, 41.03774456592552156, -130.5712005305402670 ) ) ;
#4480=EDGE_CURVE ( 'NONE', #4637, #5145, #3717, .T. ) ;
#4485=CARTESIAN_POINT ( 'NONE',  ( -975.3893330992572146, 71.12659035875115876, -95.06748246948035330 ) ) ;
#4492=CARTESIAN_POINT ( 'NONE',  ( -1023.860074334734577, 85.97273905232950142, -94.48732055948609343 ) ) ;
#4507=CARTESIAN_POINT ( 'NONE',  ( -1024.722591077092829, 118.3980260646366958, -118.7903414690678403 ) ) ;
#4521=CARTESIAN_POINT ( 'NONE',  ( -1012.226803665787770, 93.06815595962714838, -154.2940595301283224 ) ) ;
#4526=CARTESIAN_POINT ( 'NONE',  ( -927.2951026182241776, 99.13268410970675859, -154.2940595301278961 ) ) ;
#4533=CARTESIAN_POINT ( 'NONE',  ( -1038.158164256572263, 71.32123499372137587, -154.2940595301283224 ) ) ;
#4548=CARTESIAN_POINT ( 'NONE',  ( -1038.028607166439997, 78.75533988487829617, -94.48732055948607922 ) ) ;
#4552=CARTESIAN_POINT ( 'NONE',  ( -954.5692209181572707, 49.02792041507773746, -126.6442663926294045 ) ) ;
#4558=CARTESIAN_POINT ( 'NONE',  ( -1020.755281158177013, 68.40999151392674094, -99.57582448894541471 ) ) ;
#4574=CARTESIAN_POINT ( 'NONE',  ( -823.7697810748813936, 117.7733807739867871, -122.7172756069790438 ) ) ;
#4579=ADVANCED_FACE ( 'NONE', ( #7519 ), #5663, .F. ) ;
#4585=CARTESIAN_POINT ( 'NONE',  ( -1023.463303304735746, 92.47874188371233117, -154.2940595301281519 ) ) ;
#4596=CARTESIAN_POINT ( 'NONE',  ( -819.8389179520123662, 63.91331975908080665, -154.2940595301278677 ) ) ;
#4600=AXIS2_PLACEMENT_3D ( 'NONE', #4735, #10407, #11523 ) ;
#4604=CARTESIAN_POINT ( 'NONE',  ( -828.5728621739538085, 77.06309091183307203, -105.2972035265141528 ) ) ;
#4614=CARTESIAN_POINT ( 'NONE',  ( -1012.527716518103489, 86.38194213450553605, -94.48732055948642028 ) ) ;
#4623=CARTESIAN_POINT ( 'NONE',  ( -1025.000791045973756, 67.42844482392702332, -99.57582448894532945 ) ) ;
#4637=VERTEX_POINT ( 'NONE', #7702 ) ;
#4638=CARTESIAN_POINT ( 'NONE',  ( -1014.170783943992433, 114.7803637426472534, -107.9061927053325292 ) ) ;
#4649=CARTESIAN_POINT ( 'NONE',  ( -1011.662592067699165, 105.4443429699074244, -149.7857175106632326 ) ) ;
#4658=CARTESIAN_POINT ( 'NONE',  ( -955.6263874535649165, 86.32439835342530898, -154.8742214401227670 ) ) ;
#4676=CARTESIAN_POINT ( 'NONE',  ( -1025.000791045973756, 67.42844482392702332, -99.57582448894532945 ) ) ;
#4678=CARTESIAN_POINT ( 'NONE',  ( -998.0431609429218724, 37.14019503514174403, -126.6442663926292340 ) ) ;
#4680=CARTESIAN_POINT ( 'NONE',  ( -823.5011194091157449, 83.67446401253090471, -144.6105519893422127 ) ) ;
#4681=CARTESIAN_POINT ( 'NONE',  ( -954.1708249681001917, 122.1961423320944249, -136.2353035311976157 ) ) ;
#4688=CARTESIAN_POINT ( 'NONE',  ( -1032.391769651399727, 55.42093464310126905, -103.3307627799637487 ) ) ;
#4694=CARTESIAN_POINT ( 'NONE',  ( -852.9318753287178652, 113.3383058689773151, -107.9061927053323302 ) ) ;
#4701=CARTESIAN_POINT ( 'NONE',  ( -991.8293279264787543, 119.7328159579555091, -113.1262384684096673 ) ) ;
#4707=CARTESIAN_POINT ( 'NONE',  ( -952.9945178120615310, 87.05516224832936700, -154.8742214401229660 ) ) ;
#4711=CARTESIAN_POINT ( 'NONE',  ( -1065.000000000007731, 93.55451860843886891, -152.5758913445290830 ) ) ;
#4715=CARTESIAN_POINT ( 'NONE',  ( -1055.782959745576591, 85.17781532426890578, -154.2940595301287203 ) ) ;
#4721=CARTESIAN_POINT ( 'NONE',  ( -828.1678681009909724, 81.16376924194530318, -144.6638077543062479 ) ) ;
#4723=VERTEX_POINT ( 'NONE', #1460 ) ;
#4734=CARTESIAN_POINT ( 'NONE',  ( -996.5513353153756952, 56.29506814688433280, -99.57582448894517313 ) ) ;
#4735=CARTESIAN_POINT ( 'NONE',  ( -795.0000000000043201, 82.00000000000039790, -124.6807709998041105 ) ) ;
#4737=CARTESIAN_POINT ( 'NONE',  ( -1032.644706488202019, 45.21923725197559207, -130.5712005305405228 ) ) ;
#4738=CARTESIAN_POINT ( 'NONE',  ( -822.2160636604419324, 83.41847921025930646, -144.6308011508170352 ) ) ;
#4744=CARTESIAN_POINT ( 'NONE',  ( -1032.260242496269029, 61.00429285198274698, -99.57582448894517313 ) ) ;
#4760=CARTESIAN_POINT ( 'NONE',  ( -926.8105964072267398, 116.1567348237267083, -146.0307792196442733 ) ) ;
#4769=CARTESIAN_POINT ( 'NONE',  ( -1017.840614713428863, 119.3387310954208118, -130.5712005305402954 ) ) ;
#4778=CARTESIAN_POINT ( 'NONE',  ( -1024.641217300042399, 73.20632742167555307, -152.5758913445296230 ) ) ;
#4790=CARTESIAN_POINT ( 'NONE',  ( -1032.113539130918525, 67.34854938887495734, -96.78565065507952170 ) ) ;
#4791=CARTESIAN_POINT ( 'NONE',  ( -828.8285638327243987, 78.67432280806561096, -104.9592124606052863 ) ) ;
#4799=CARTESIAN_POINT ( 'NONE',  ( -1062.923339974269538, 49.86928741160662071, -113.1262384684094968 ) ) ;
#4809=ORIENTED_EDGE ( 'NONE', *, *, #2065, .T. ) ;
#4811=CARTESIAN_POINT ( 'NONE',  ( -1024.722591077094876, 118.3980260646368379, -130.5712005305404944 ) ) ;
#4814=CARTESIAN_POINT ( 'NONE',  ( -1065.000000000003411, 111.6133447792289104, -118.7903414690678972 ) ) ;
#4824=CARTESIAN_POINT ( 'NONE',  ( -1025.296800000958683, 108.9225844456048691, -146.0307792196446144 ) ) ;
#4832=CARTESIAN_POINT ( 'NONE',  ( -795.0000000000002274, 56.89504896194490868, -141.4553492942756350 ) ) ;
#4842=CARTESIAN_POINT ( 'NONE',  ( -853.8938961404153360, 37.86297855175766358, -103.3307627799636776 ) ) ;
#4851=CARTESIAN_POINT ( 'NONE',  ( -1017.027421246622112, 56.01181809833683900, -113.1262384684095537 ) ) ;
#4856=CARTESIAN_POINT ( 'NONE',  ( -1060.958858734054957, 107.4804882715807963, -107.9061927053325007 ) ) ;
#4861=CARTESIAN_POINT ( 'NONE',  ( -951.7027691703317487, 118.7449601027236241, -107.9061927053324581 ) ) ;
#4867=CARTESIAN_POINT ( 'NONE',  ( -926.5138833012647410, 125.7648744980332225, -124.6807709998040394 ) ) ;
#4869=AXIS2_PLACEMENT_3D ( 'NONE', #12031, #11103, #1778 ) ;
#4876=CARTESIAN_POINT ( 'NONE',  ( -1037.337636019037518, 116.9882293220590270, -126.6442663926289640 ) ) ;
#4887=CARTESIAN_POINT ( 'NONE',  ( -1057.036663358150690, 58.23757105449725913, -149.7857175106634884 ) ) ;
#4893=CARTESIAN_POINT ( 'NONE',  ( -1014.004070199769671, 54.58258344709567922, -136.2353035311988947 ) ) ;
#4900=CARTESIAN_POINT ( 'NONE',  ( -1032.503061859599256, 50.81309391744463255, -107.9061927053326428 ) ) ;
#4908=VECTOR ( 'NONE', #11616, 1000.000000000000000 ) ;
#4911=CARTESIAN_POINT ( 'NONE',  ( -957.0819499390169085, 50.45265437475560333, -113.1262384684095537 ) ) ;
#4925=CARTESIAN_POINT ( 'NONE',  ( -955.0423082396529253, 101.0797422464698059, -96.78565065507901011 ) ) ;
#4926=CARTESIAN_POINT ( 'NONE',  ( -954.1708249681001917, 122.1961423320944249, -136.2353035311976157 ) ) ;
#4929=CARTESIAN_POINT ( 'NONE',  ( -1021.743962174751232, 119.2557508373789403, -124.6807709998040110 ) ) ;
#4935=CARTESIAN_POINT ( 'NONE',  ( -1031.086615573508880, 111.8776252365151009, -141.4553492942759760 ) ) ;
#4936=CARTESIAN_POINT ( 'NONE',  ( -818.8285638327243987, 78.67432280806558254, -94.73795703228648790 ) ) ;
#4941=CARTESIAN_POINT ( 'NONE',  ( -904.2101318205999405, 125.2895275102983419, -124.6807709998041531 ) ) ;
#4943=CARTESIAN_POINT ( 'NONE',  ( -1037.461794897090840, 110.6138330393710731, -141.4553492942763171 ) ) ;
#4948=CARTESIAN_POINT ( 'NONE',  ( -820.7525053003688527, 74.71879621637260982, -106.0522004026988867 ) ) ;
#4949=CARTESIAN_POINT ( 'NONE',  ( -902.0880155070129831, 62.23309906011792947, -141.4553492942754644 ) ) ;
#4957=CARTESIAN_POINT ( 'NONE',  ( -1017.133222628203043, 54.07990892584120246, -130.5712005305404375 ) ) ;
#4962=CARTESIAN_POINT ( 'NONE',  ( -1017.133222628208614, 54.07990892584129483, -118.7903414690683519 ) ) ;
#4972=CARTESIAN_POINT ( 'NONE',  ( -854.0393178910176175, 26.93106345811105840, -113.1262384684097100 ) ) ;
#4975=CARTESIAN_POINT ( 'NONE',  ( -1037.773541645229670, 93.34895244571353601, -96.78565065507908116 ) ) ;
#4979=CARTESIAN_POINT ( 'NONE',  ( -955.0000000000038654, 82.00000000000036948, -124.6807709998041673 ) ) ;
#4981=CARTESIAN_POINT ( 'NONE',  ( -955.3297122972882107, 93.84065249268854814, -95.06748246948001224 ) ) ;
#4983=CARTESIAN_POINT ( 'NONE',  ( -852.9318753287220716, 113.3383058689776277, -141.4553492942764024 ) ) ;
#4986=CARTESIAN_POINT ( 'NONE',  ( -974.1288507787422759, 124.2142274477005657, -124.6807709998040110 ) ) ;
#4989=AXIS2_PLACEMENT_3D ( 'NONE', #7521, #12223, #10242 ) ;
#4992=CARTESIAN_POINT ( 'NONE',  ( -1025.296800000958683, 108.9225844456048691, -146.0307792196446144 ) ) ;
#5000=CARTESIAN_POINT ( 'NONE',  ( -795.0000000000006821, 98.77454568802552615, -149.7857175106634884 ) ) ;
#5006=CARTESIAN_POINT ( 'NONE',  ( -996.0013826475917540, 63.70094029248592449, -152.5758913445294240 ) ) ;
#5020=CARTESIAN_POINT ( 'NONE',  ( -901.8967518049364571, 57.00804855647901093, -118.7903414690679540 ) ) ;
#5022=ORIENTED_EDGE ( 'NONE', *, *, #7195, .T. ) ;
#5031=CARTESIAN_POINT ( 'NONE',  ( -817.1493800258448346, 27.50875274330015685, -122.7172756069792001 ) ) ;
#5036=CARTESIAN_POINT ( 'NONE',  ( -954.7734463792770612, 107.7731650919851205, -99.57582448894495997 ) ) ;
#5041=CARTESIAN_POINT ( 'NONE',  ( -794.9999999999997726, 87.89043812168591785, -95.06748246948019698 ) ) ;
#5044=CARTESIAN_POINT ( 'NONE',  ( -904.1167769183923610, 122.8348148996190758, -136.2353035311977862 ) ) ;
#5055=FACE_OUTER_BOUND ( 'NONE', #3199, .T. ) ;
#5056=FACE_OUTER_BOUND ( 'NONE', #5512, .T. ) ;
#5058=CARTESIAN_POINT ( 'NONE',  ( -1022.396981161619806, 109.5926079579672603, -146.0307792196444154 ) ) ;
#5065=CARTESIAN_POINT ( 'NONE',  ( -795.0000000000071623, 70.44548139156209743, -152.5758913445292535 ) ) ;
#5080=CARTESIAN_POINT ( 'NONE',  ( -1057.805062346511704, 42.77845103615958067, -118.7903414690684087 ) ) ;
#5083=ORIENTED_EDGE ( 'NONE', *, *, #12205, .F. ) ;
#5084=CARTESIAN_POINT ( 'NONE',  ( -818.9871366297778650, 79.96561131121026733, -144.5796535119517614 ) ) ;
#5091=CARTESIAN_POINT ( 'NONE',  ( -817.4144546772188278, 30.82543593413045713, -113.1262384684093689 ) ) ;
#5097=CARTESIAN_POINT ( 'NONE',  ( -1018.401127491270358, 110.2021201405460431, -103.3307627799636208 ) ) ;
#5104=EDGE_CURVE ( 'NONE', #8436, #11949, #5357, .T. ) ;
#5106=CARTESIAN_POINT ( 'NONE',  ( -1061.884876827091830, 80.20192378191423188, -94.48732055948617869 ) ) ;
#5109=CARTESIAN_POINT ( 'NONE',  ( -1017.810720698609543, 119.7719591276204625, -124.6807709998040679 ) ) ;
#5114=CARTESIAN_POINT ( 'NONE',  ( -1031.000617048998265, 115.3267894020684992, -113.1262384684098521 ) ) ;
#5117=B_SPLINE_CURVE_WITH_KNOTS ( 'NONE', 3,
 ( #1549, #8847, #3162, #6188, #2239, #9082, #6251, #7112, #374, #11700, #10018, #6066, #10876, #8896, #4099, #557, #11870, #5311, #3213, #2411, #1370, #2361, #9959, #7870, #6007, #5248, #4212, #1315, #6128, #9895, #4337, #3644, #5506, #4460, #3455, #2595 ),
 .UNSPECIFIED., .F., .F.,
 ( 4, 2, 2, 2, 2, 2, 2, 2, 2, 2, 2, 2, 2, 2, 2, 2, 2, 4 ),
 ( 0.01566740727309163389, 0.01664433654934411103, 0.01762126582559659163, 0.01859819510184906877, 0.01957512437810154590, 0.02055205365435402304, 0.02152898293060650364, 0.02250591220685898078, 0.02348284148311145791, 0.02445977075936393852, 0.02494823539749017882, 0.02543670003561641565, 0.02641362931186860483, 0.02739055858812079053, 0.02836748786437297970, 0.02934441714062516887, 0.03032134641687735804, 0.03129827569312954721 ),
 .UNSPECIFIED. ) ;
#5127=CARTESIAN_POINT ( 'NONE',  ( -1030.931480980267906, 117.9615145441170654, -124.6807709998043521 ) ) ;
#5138=CARTESIAN_POINT ( 'NONE',  ( -1027.708477481189902, 65.70736702952426356, -149.7857175106639431 ) ) ;
#5142=CARTESIAN_POINT ( 'NONE',  ( -1064.999999999999545, 54.10491585757062438, -113.1262384684097668 ) ) ;
#5144=CARTESIAN_POINT ( 'NONE',  ( -824.4843289719594850, 83.64195140549487917, -95.25604041866178306 ) ) ;
#5145=VERTEX_POINT ( 'NONE', #10123 ) ;
#5148=ORIENTED_EDGE ( 'NONE', *, *, #2970, .F. ) ;
#5153=CARTESIAN_POINT ( 'NONE',  ( -955.0423082396529253, 101.0797422464698059, -96.78565065507901011 ) ) ;
#5164=CARTESIAN_POINT ( 'NONE',  ( -1026.284439350007460, 91.37828661775220951, -95.06748246948018277 ) ) ;
#5166=CARTESIAN_POINT ( 'NONE',  ( -1037.337636019038882, 116.9882293220588991, -124.6807709998043521 ) ) ;
#5173=CARTESIAN_POINT ( 'NONE',  ( -1025.976186494711783, 52.68972726728017619, -124.6807709998042952 ) ) ;
#5174=CARTESIAN_POINT ( 'NONE',  ( -820.7733255381026538, 82.64589962596730288, -95.09174178707476699 ) ) ;
#5179=CARTESIAN_POINT ( 'NONE',  ( -1017.810720698609543, 119.7719591276204625, -124.6807709998040679 ) ) ;
#5192=CARTESIAN_POINT ( 'NONE',  ( -902.2382941300837729, 66.55116351576596401, -146.0307792196448986 ) ) ;
#5196=CARTESIAN_POINT ( 'NONE',  ( -997.9925905826713688, 37.72784750336357007, -118.7903414690684514 ) ) ;
#5205=CARTESIAN_POINT ( 'NONE',  ( -1065.000000000008868, 103.3499740386314016, -103.3307627799635924 ) ) ;
#5216=CARTESIAN_POINT ( 'NONE',  ( -795.0000000000047748, 112.0000000000007532, -124.6807709998042384 ) ) ;
#5219=CARTESIAN_POINT ( 'NONE',  ( -1016.123300349496276, 74.17810748283143596, -96.78565065507957854 ) ) ;
#5221=CARTESIAN_POINT ( 'NONE',  ( -926.5138833012656505, 125.7648744980332225, -126.6442663926294330 ) ) ;
#5228=CARTESIAN_POINT ( 'NONE',  ( -954.5692209181579528, 49.02792041507773746, -124.6807709998042384 ) ) ;
#5230=CARTESIAN_POINT ( 'NONE',  ( -821.3191871189538915, 83.01147993754599952, -95.14350462154642685 ) ) ;
#5234=CARTESIAN_POINT ( 'NONE',  ( -852.8175266017511831, 121.6828083272127685, -124.6807709998041247 ) ) ;
#5238=CARTESIAN_POINT ( 'NONE',  ( -993.6119331254993767, 96.30709745136249467, -152.5758913445288840 ) ) ;
#5248=CARTESIAN_POINT ( 'NONE',  ( -820.7839104893611193, 74.69477923707955824, -94.69500076520461107 ) ) ;
#5252=CARTESIAN_POINT ( 'NONE',  ( -795.0000000000039790, 54.10491585757074517, -136.2353035311982410 ) ) ;
#5270=CARTESIAN_POINT ( 'NONE',  ( -794.9999999999997726, 87.89043812168591785, -95.06748246948019698 ) ) ;
#5279=CARTESIAN_POINT ( 'NONE',  ( -827.1386055644237558, 82.43593308702942579, -154.2518061096776876 ) ) ;
#5280=CARTESIAN_POINT ( 'NONE',  ( -853.4539021257702416, 72.48584973915980356, -94.48732055948642028 ) ) ;
#5288=CARTESIAN_POINT ( 'NONE',  ( -1038.719578313838156, 40.52245044769760085, -124.6807709998045652 ) ) ;
#5291=CARTESIAN_POINT ( 'NONE',  ( -954.0441199534440102, 124.9954171138387977, -124.6807709998039115 ) ) ;
#5305=CARTESIAN_POINT ( 'NONE',  ( -953.2897746444480163, 79.65961628290892804, -154.2940595301281519 ) ) ;
#5309=CARTESIAN_POINT ( 'NONE',  ( -955.0000000000038654, 82.00000000000036948, -124.6807709998041673 ) ) ;
#5311=CARTESIAN_POINT ( 'NONE',  ( -823.5029313004960159, 73.67403370300826282, -94.71553284777590420 ) ) ;
#5316=CARTESIAN_POINT ( 'NONE',  ( -1048.040919118598822, 50.77060569800413248, -146.0307792196448986 ) ) ;
#5333=CARTESIAN_POINT ( 'NONE',  ( -1062.096538105501168, 73.81465972843167833, -95.06748246948046699 ) ) ;
#5342=CARTESIAN_POINT ( 'NONE',  ( -1065.000000000001364, 70.44548139156162847, -96.78565065507940801 ) ) ;
#5350=CARTESIAN_POINT ( 'NONE',  ( -819.4886076266410555, 76.16999570164527711, -154.6813788771335680 ) ) ;
#5353=CARTESIAN_POINT ( 'NONE',  ( -1030.944970944895431, 117.4714819019837222, -118.7903414690680535 ) ) ;
#5357=CIRCLE ( 'NONE', #2604, 30.00000000000021316 ) ;
#5362=CARTESIAN_POINT ( 'NONE',  ( -1012.527716518106786, 86.38194213450564973, -154.8742214401233070 ) ) ;
#5374=CARTESIAN_POINT ( 'NONE',  ( -928.2641150402240555, 65.00826535581498433, -141.4553492942759476 ) ) ;
#5387=CARTESIAN_POINT ( 'NONE',  ( -1017.158871447983074, 53.64146012065780411, -126.6442663926291061 ) ) ;
#5392=CARTESIAN_POINT ( 'NONE',  ( -818.8610518734294601, 79.33190776187021243, -154.5898210126322851 ) ) ;
#5393=CARTESIAN_POINT ( 'NONE',  ( -795.0000000000080718, 82.00000000000049738, -94.48732055948593711 ) ) ;
#5414=CYLINDRICAL_SURFACE ( 'NONE', #11580, 5.000000000000115463 ) ;
#5415=CARTESIAN_POINT ( 'NONE',  ( -1054.380968608932108, 114.0683136310379524, -122.7172756069792570 ) ) ;
#5428=CARTESIAN_POINT ( 'NONE',  ( -1015.517346982278013, 86.95624952299075971, -154.8742214401231649 ) ) ;
#5429=CARTESIAN_POINT ( 'NONE',  ( -826.0729559276804821, 74.19411019796237383, -143.0951037527842686 ) ) ;
#5437=CARTESIAN_POINT ( 'NONE',  ( -1056.743458481019616, 64.45745743522664384, -152.5758913445293956 ) ) ;
#5458=CARTESIAN_POINT ( 'NONE',  ( -994.1998135634719347, 88.30642396300639518, -95.06748246948001224 ) ) ;
#5461=CARTESIAN_POINT ( 'NONE',  ( -1048.438004920982848, 39.66697241395321782, -126.6442663926296603 ) ) ;
#5462=CARTESIAN_POINT ( 'NONE',  ( -824.1603064692830003, 83.67418067986891117, -144.6105757924098327 ) ) ;
#5469=CARTESIAN_POINT ( 'NONE',  ( -1047.151245865161172, 77.61790247226321071, -94.48732055948626396 ) ) ;
#5484=CARTESIAN_POINT ( 'NONE',  ( -818.8609295919769693, 78.01955378747423708, -154.6506939777316632 ) ) ;
#5487=CARTESIAN_POINT ( 'NONE',  ( -954.0441199534441239, 124.9954171138387977, -122.7172756069788875 ) ) ;
#5501=CARTESIAN_POINT ( 'NONE',  ( -1037.656130532295037, 99.96792753513321372, -149.7857175106633747 ) ) ;
#5506=CARTESIAN_POINT ( 'NONE',  ( -818.9900958282657939, 77.37130366011599847, -94.69300966023514832 ) ) ;
#5510=CARTESIAN_POINT ( 'NONE',  ( -995.4135022096103285, 71.70161378084171133, -154.2940595301282656 ) ) ;
#5512=EDGE_LOOP ( 'NONE', ( #9203, #5699, #4179, #10085 ) ) ;
#5526=CARTESIAN_POINT ( 'NONE',  ( -1026.651933061283898, 84.71212313386838844, -94.48732055948616448 ) ) ;
#5528=CARTESIAN_POINT ( 'NONE',  ( -1065.000000000000682, 52.38665522077219805, -130.5712005305403238 ) ) ;
#5529=CARTESIAN_POINT ( 'NONE',  ( -820.0597211274506435, 81.97619047958284000, -144.6820902952100596 ) ) ;
#5537=CARTESIAN_POINT ( 'NONE',  ( -1016.652307257391612, 63.31440937415304404, -103.3307627799640045 ) ) ;
#5552=CARTESIAN_POINT ( 'NONE',  ( -1045.967528061859412, 112.8272211019270230, -113.1262384684098663 ) ) ;
#5561=CARTESIAN_POINT ( 'NONE',  ( -974.7984820115178763, 96.63273410478066694, -152.5758913445288272 ) ) ;
#5564=CARTESIAN_POINT ( 'NONE',  ( -1055.469533842436022, 91.91071092603651493, -152.5758913445291398 ) ) ;
#5570=CARTESIAN_POINT ( 'NONE',  ( -953.5758047008371250, 72.53746257253824581, -152.5758913445294525 ) ) ;
#5574=EDGE_LOOP ( 'NONE', ( #9149, #3446, #8240, #3269 ) ) ;
#5577=CARTESIAN_POINT ( 'NONE',  ( -828.8285638327246261, 78.99577924834096621, -144.4565372401591219 ) ) ;
#5579=CARTESIAN_POINT ( 'NONE',  ( -828.7963533401381255, 78.01901522663844446, -105.0781937692942734 ) ) ;
#5589=CARTESIAN_POINT ( 'NONE',  ( -997.0443963278638648, 49.75991663364290929, -103.3307627799637487 ) ) ;
#5592=CARTESIAN_POINT ( 'NONE',  ( -957.2086549536780922, 47.65337959301152893, -122.7172756069790012 ) ) ;
#5593=CARTESIAN_POINT ( 'NONE',  ( -824.4888212380200230, 83.64126188030940057, -144.6134169528915265 ) ) ;
#5599=CARTESIAN_POINT ( 'NONE',  ( -1057.521967982379238, 48.25222617154000204, -107.9061927053324723 ) ) ;
#5604=CARTESIAN_POINT ( 'NONE',  ( -1025.044148074454370, 113.2108726315405960, -107.9061927053325007 ) ) ;
#5621=CARTESIAN_POINT ( 'NONE',  ( -853.2189900670995257, 91.12674563889149226, -152.5758913445289693 ) ) ;
#5626=CARTESIAN_POINT ( 'NONE',  ( -1061.468168685229102, 92.73456844357778550, -152.5758913445291398 ) ) ;
#5633=CARTESIAN_POINT ( 'NONE',  ( -1047.151245865163673, 77.61790247226322492, -154.8742214401233070 ) ) ;
#5634=CARTESIAN_POINT ( 'NONE',  ( -1054.380968608929606, 114.0683136310380803, -126.6442663926291345 ) ) ;
#5639=CARTESIAN_POINT ( 'NONE',  ( -826.9035580924005444, 74.71835857218601973, -106.0523996049648474 ) ) ;
#5641=CARTESIAN_POINT ( 'NONE',  ( -1021.293373424891683, 59.24127555818969171, -141.4553492942756918 ) ) ;
#5649=EDGE_CURVE ( 'NONE', #1185, #915, #10707, .T. ) ;
#5652=CARTESIAN_POINT ( 'NONE',  ( -853.6888141844383426, 53.84495383942796565, -96.78565065507952170 ) ) ;
#5653=CARTESIAN_POINT ( 'NONE',  ( -821.3208927675284485, 83.01261617298027318, -104.7055743826754224 ) ) ;
#5654=CARTESIAN_POINT ( 'NONE',  ( -817.1493800258448346, 27.50875274330015685, -122.7172756069792001 ) ) ;
#5662=CARTESIAN_POINT ( 'NONE',  ( -997.4616017999825317, 44.34671234275855767, -107.9061927053325007 ) ) ;
#5663=CYLINDRICAL_SURFACE ( 'NONE', #11422, 5.000000000000115463 ) ;
#5673=CARTESIAN_POINT ( 'NONE',  ( -1031.086615573502741, 111.8776252365149730, -107.9061927053324723 ) ) ;
#5680=CARTESIAN_POINT ( 'NONE',  ( -1054.913455627173789, 103.6024512377076974, -146.0307792196445291 ) ) ;
#5683=DIRECTION ( 'NONE',  ( 0.000000000000000000, 5.522905491341382306E-16, 1.000000000000000000 ) ) ;
#5687=CARTESIAN_POINT ( 'NONE',  ( -975.5821371384174654, 62.83201726680850641, -152.5758913445291682 ) ) ;
#5696=CARTESIAN_POINT ( 'NONE',  ( -827.6030183929074155, 81.96987526947719971, -144.6820941065185195 ) ) ;
#5698=CARTESIAN_POINT ( 'NONE',  ( -854.0393178910245524, 26.93106345811121827, -136.2353035311989515 ) ) ;
#5699=ORIENTED_EDGE ( 'NONE', *, *, #3479, .T. ) ;
#5708=CARTESIAN_POINT ( 'NONE',  ( -902.4158961391592584, 71.79205886009090420, -99.57582448894511629 ) ) ;
#5720=CARTESIAN_POINT ( 'NONE',  ( -795.0000000000070486, 70.44548139156158584, -96.78565065507937959 ) ) ;
#5724=CARTESIAN_POINT ( 'NONE',  ( -823.5047064235060361, 114.4566975831561848, -113.1262384684095537 ) ) ;
#5731=CARTESIAN_POINT ( 'NONE',  ( -951.9057582426089539, 113.9552214607315364, -103.3307627799633082 ) ) ;
#5732=B_SPLINE_CURVE_WITH_KNOTS ( 'NONE', 3,
 ( #10576, #5577, #9350, #7496, #1875, #9468, #6684, #4721, #12201, #1933, #5696, #3721, #1769, #3862, #19, #2619, #2686, #5593, #5462, #4680, #11095, #12215, #4738, #3739, #1951, #6459, #779, #8328, #9304, #5529, #1892, #7753, #8626, #7694, #5084, #10477, #2134, #2074 ),
 .UNSPECIFIED., .F., .F.,
 ( 4, 2, 2, 2, 2, 2, 2, 2, 2, 2, 2, 2, 2, 2, 2, 2, 2, 2, 4 ),
 ( 0.01596000347429179719, 0.01693787742768236571, 0.01791575138107293769, 0.01840468835776813694, 0.01889362533446333967, 0.01987149928785374858, 0.02084937324124415403, 0.02182724719463455948, 0.02280512114802496493, 0.02378299510141537038, 0.02476086905480577582, 0.02573874300819618474, 0.02671661696158659019, 0.02720555393828179291, 0.02769449091497699564, 0.02867236486836743231, 0.02965023882175786898, 0.03062811277514830566, 0.03160598672853873886 ),
 .UNSPECIFIED. ) ;
#5734=CARTESIAN_POINT ( 'NONE',  ( -1060.846413679901389, 110.5345601522218146, -136.2353035311979852 ) ) ;
#5740=CARTESIAN_POINT ( 'NONE',  ( -795.0000000000021600, 107.1049510380564129, -141.4553492942762318 ) ) ;
#5747=CARTESIAN_POINT ( 'NONE',  ( -1046.095701327183860, 109.2451008237763546, -141.4553492942764308 ) ) ;
#5749=ORIENTED_EDGE ( 'NONE', *, *, #8881, .T. ) ;
#5754=CARTESIAN_POINT ( 'NONE',  ( -1062.665377791219498, 57.01990411978283646, -146.0307792196448702 ) ) ;
#5759=FILL_AREA_STYLE_COLOUR ( '', #1341 ) ;
#5764=CARTESIAN_POINT ( 'NONE',  ( -1057.036663358159558, 58.23757105449750071, -99.57582448894497418 ) ) ;
#5765=CARTESIAN_POINT ( 'NONE',  ( -1065.000000000006366, 82.00000000000036948, -124.6807709998044231 ) ) ;
#5775=CARTESIAN_POINT ( 'NONE',  ( -1025.943122242217214, 53.12767954719360830, -118.7903414690682524 ) ) ;
#5778=CARTESIAN_POINT ( 'NONE',  ( -1046.095701327177267, 109.2451008237761982, -107.9061927053324439 ) ) ;
#5785=CARTESIAN_POINT ( 'NONE',  ( -823.5047064235060361, 114.4566975831561848, -113.1262384684095537 ) ) ;
#5786=CARTESIAN_POINT ( 'NONE',  ( -1017.963927524549604, 117.4283576114808625, -136.2353035311979284 ) ) ;
#5791=CARTESIAN_POINT ( 'NONE',  ( -926.5138833012644000, 125.7648744980332225, -122.7172756069789159 ) ) ;
#5793=CARTESIAN_POINT ( 'NONE',  ( -951.4198147059589701, 125.0824040815807194, -124.6807709998040252 ) ) ;
#5796=CARTESIAN_POINT ( 'NONE',  ( -853.1108559448500728, 99.60875591605696400, -149.7857175106632610 ) ) ;
#5806=CARTESIAN_POINT ( 'NONE',  ( -974.6181169426273527, 104.3135445892218200, -149.7857175106634884 ) ) ;
#5809=VERTEX_POINT ( 'NONE', #433 ) ;
#5812=CARTESIAN_POINT ( 'NONE',  ( -818.8614508132119454, 78.01542073698772128, -105.0789755614320029 ) ) ;
#5814=CARTESIAN_POINT ( 'NONE',  ( -818.1708872189602744, 40.82851623284160070, -146.0307792196448702 ) ) ;
#5827=CARTESIAN_POINT ( 'NONE',  ( -1065.000000000002501, 60.65002596136933732, -103.3307627799636350 ) ) ;
#5828=CARTESIAN_POINT ( 'NONE',  ( -795.0000000000043201, 62.00000000000031974, -124.6807709998041815 ) ) ;
#5829=CARTESIAN_POINT ( 'NONE',  ( -854.0803342822151762, 23.97549884981696167, -130.5712005305403238 ) ) ;
#5838=CARTESIAN_POINT ( 'NONE',  ( -928.4218612484631876, 59.99049470396640515, -118.7903414690680535 ) ) ;
#5844=CARTESIAN_POINT ( 'NONE',  ( -1065.000000000000455, 107.1049510380560719, -107.9061927053323302 ) ) ;
#5850=CARTESIAN_POINT ( 'NONE',  ( -926.9570750291553622, 111.1083136274928620, -99.57582448894491733 ) ) ;
#5854=CARTESIAN_POINT ( 'NONE',  ( -1030.931480980267906, 117.9615145441170654, -124.6807709998043521 ) ) ;
#5859=CARTESIAN_POINT ( 'NONE',  ( -974.4564103291385209, 111.0951925441807759, -146.0307792196441312 ) ) ;
#5867=CARTESIAN_POINT ( 'NONE',  ( -1046.261572611719657, 104.4651992465226868, -146.0307792196445575 ) ) ;
#5875=CARTESIAN_POINT ( 'NONE',  ( -1027.375436305353333, 71.63039521860234515, -152.5758913445296230 ) ) ;
#5877=( GEOMETRIC_REPRESENTATION_CONTEXT ( 3 ) GLOBAL_UNCERTAINTY_ASSIGNED_CONTEXT ( ( #5967 ) ) GLOBAL_UNIT_ASSIGNED_CONTEXT ( ( #8733, #7049, #375 ) ) REPRESENTATION_CONTEXT ( 'NONE', 'WORKASPACE' ) );
#5889=CARTESIAN_POINT ( 'NONE',  ( -1032.589060384100776, 47.36392975189028931, -113.1262384684095537 ) ) ;
#5890=CARTESIAN_POINT ( 'NONE',  ( -828.5765974139392256, 80.27527354417625816, -104.7529721962251585 ) ) ;
#5892=CARTESIAN_POINT ( 'NONE',  ( -1025.806732200655688, 55.05754055295027172, -136.2353035311988663 ) ) ;
#5905=CARTESIAN_POINT ( 'NONE',  ( -901.9718911164643487, 59.00785292138902349, -113.1262384684096105 ) ) ;
#5909=CARTESIAN_POINT ( 'NONE',  ( -1025.595388641369482, 103.7168792382126128, -99.57582448894517313 ) ) ;
#5917=ORIENTED_EDGE ( 'NONE', *, *, #9611, .T. ) ;
#5918=CARTESIAN_POINT ( 'NONE',  ( -1014.911393615048723, 99.73439156314999821, -96.78565065507932275 ) ) ;
#5919=VERTEX_POINT ( 'NONE', #7378 ) ;
#5922=CARTESIAN_POINT ( 'NONE',  ( -991.5701548301638013, 122.8678427087060214, -122.7172756069787170 ) ) ;
#5927=CARTESIAN_POINT ( 'NONE',  ( -1054.691024341075263, 108.1159421897237962, -141.4553492942763739 ) ) ;
#5935=CARTESIAN_POINT ( 'NONE',  ( -1054.913455627173789, 103.6024512377076974, -146.0307792196445291 ) ) ;
#5938=ORIENTED_EDGE ( 'NONE', *, *, #7308, .F. ) ;
#5941=CARTESIAN_POINT ( 'NONE',  ( -1056.743458481019616, 64.45745743522664384, -152.5758913445293956 ) ) ;
#5942=CARTESIAN_POINT ( 'NONE',  ( -819.3325619471245318, 76.46264315494626373, -143.9014485902362708 ) ) ;
#5954=CARTESIAN_POINT ( 'NONE',  ( -1048.417899310738221, 40.17786091688638095, -118.7903414690680250 ) ) ;
#5957=CARTESIAN_POINT ( 'NONE',  ( -817.2011019090375612, 28.13185037056175375, -130.5712005305403238 ) ) ;
#5965=CARTESIAN_POINT ( 'NONE',  ( -1048.334963668458158, 42.40858384259915681, -113.1262384684096105 ) ) ;
#5967=UNCERTAINTY_MEASURE_WITH_UNIT (LENGTH_MEASURE( 1.000000000000000082E-05 ), #8733, 'distance_accuracy_value', 'NONE');
#5968=CARTESIAN_POINT ( 'NONE',  ( -993.0619804577127070, 103.7129695969639442, -99.57582448894480365 ) ) ;
#5975=CARTESIAN_POINT ( 'NONE',  ( -853.2189900670988436, 91.12674563889150647, -96.78565065507912379 ) ) ;
#5976=CARTESIAN_POINT ( 'NONE',  ( -852.8274699693135972, 120.9962006285028906, -130.5712005305406933 ) ) ;
#5977=CARTESIAN_POINT ( 'NONE',  ( -955.0000000000038654, 62.00000000000029132, -124.6807709998041815 ) ) ;
#5991=CARTESIAN_POINT ( 'NONE',  ( -951.7027691703365235, 118.7449601027238799, -141.4553492942759192 ) ) ;
#6000=CARTESIAN_POINT ( 'NONE',  ( -1013.120138696094841, 73.26074010992857666, -152.5758913445291682 ) ) ;
#6007=CARTESIAN_POINT ( 'NONE',  ( -821.3274957761739188, 74.33250986977238028, -94.70253061673973605 ) ) ;
#6010=CARTESIAN_POINT ( 'NONE',  ( -928.3598895238005753, 61.90886769853032945, -136.2353035311983263 ) ) ;
#6015=CARTESIAN_POINT ( 'NONE',  ( -1057.832023714519210, 42.29985473022490794, -122.7172756069794559 ) ) ;
#6018=CARTESIAN_POINT ( 'NONE',  ( -1017.027421246632343, 56.01181809833700243, -136.2353035311990368 ) ) ;
#6028=CARTESIAN_POINT ( 'NONE',  ( -997.9925905826713688, 37.72784750336357007, -118.7903414690684514 ) ) ;
#6033=CARTESIAN_POINT ( 'NONE',  ( -951.9057582426089539, 113.9552214607315364, -103.3307627799633082 ) ) ;
#6038=CARTESIAN_POINT ( 'NONE',  ( -795.0000000000079581, 93.55451860843940892, -96.78565065507920906 ) ) ;
#6040=CARTESIAN_POINT ( 'NONE',  ( -852.8175266017517515, 121.6828083272129106, -126.6442663926292624 ) ) ;
#6047=CARTESIAN_POINT ( 'NONE',  ( -1057.832023714519664, 42.29985473022490794, -124.6807709998044373 ) ) ;
#6054=PRODUCT_DEFINITION_SHAPE ( 'NONE', 'NONE',  #11540 ) ;
#6060=CARTESIAN_POINT ( 'NONE',  ( -1023.860074334738101, 85.97273905232952984, -154.8742214401228523 ) ) ;
#6061=CARTESIAN_POINT ( 'NONE',  ( -821.2963138009687327, 74.35985007445715667, -143.1641509997129731 ) ) ;
#6066=CARTESIAN_POINT ( 'NONE',  ( -826.3364923082716587, 74.33644497882033875, -94.69033226336712517 ) ) ;
#6071=CARTESIAN_POINT ( 'NONE',  ( -1013.637332661010191, 62.09754518945636903, -146.0307792196449839 ) ) ;
#6077=CARTESIAN_POINT ( 'NONE',  ( -1038.708781889661850, 41.03774456592562103, -118.7903414690682240 ) ) ;
#6086=CARTESIAN_POINT ( 'NONE',  ( -854.0902776497797504, 23.28889115110667518, -126.6442663926296603 ) ) ;
#6092=CARTESIAN_POINT ( 'NONE',  ( -974.7984820115178763, 96.63273410478059589, -96.78565065507896747 ) ) ;
#6101=CARTESIAN_POINT ( 'NONE',  ( -1065.000000000004093, 93.55451860843899681, -96.78565065507908116 ) ) ;
#6104=CARTESIAN_POINT ( 'NONE',  ( -926.5289067496701136, 125.3297071905304989, -130.5712005305407786 ) ) ;
#6107=CARTESIAN_POINT ( 'NONE',  ( -1017.963927524554038, 117.4283576114806777, -113.1262384684094968 ) ) ;
#6115=CARTESIAN_POINT ( 'NONE',  ( -819.8508737614558868, 81.72136211720568610, -94.97649986144543277 ) ) ;
#6119=CARTESIAN_POINT ( 'NONE',  ( -852.8175266017511831, 121.6828083272127685, -124.6807709998041247 ) ) ;
#6128=CARTESIAN_POINT ( 'NONE',  ( -819.8574495259266541, 75.61847659506229036, -94.68200740722480191 ) ) ;
#6131=CARTESIAN_POINT ( 'NONE',  ( -902.0880155070129831, 62.23309906011792947, -141.4553492942754644 ) ) ;
#6136=CARTESIAN_POINT ( 'NONE',  ( -1038.719578313838610, 40.52245044769760085, -122.7172756069793707 ) ) ;
#6147=CARTESIAN_POINT ( 'NONE',  ( -1055.782959745578182, 85.17781532426863578, -95.06748246948041015 ) ) ;
#6155=ORIENTED_EDGE ( 'NONE', *, *, #10410, .F. ) ;
#6158=CARTESIAN_POINT ( 'NONE',  ( -819.8389179520128209, 63.91331975908082086, -95.06748246948014014 ) ) ;
#6160=CARTESIAN_POINT ( 'NONE',  ( -1054.380968608931425, 114.0683136310379524, -124.6807709998043663 ) ) ;
#6176=CARTESIAN_POINT ( 'NONE',  ( -1024.691966601152672, 118.8493250655916142, -124.6807709998039400 ) ) ;
#6184=CARTESIAN_POINT ( 'NONE',  ( -902.8257469293334907, 84.21185948885708683, -154.2940595301280950 ) ) ;
#6188=CARTESIAN_POINT ( 'NONE',  ( -828.6693929326720536, 77.38039550993836713, -94.71761797639442193 ) ) ;
#6193=CARTESIAN_POINT ( 'NONE',  ( -1048.206790403134164, 45.99070412075050740, -141.4553492942756918 ) ) ;
#6211=CARTESIAN_POINT ( 'NONE',  ( -1031.794838716553841, 81.34535957697958963, -94.48732055948609343 ) ) ;
#6213=SHAPE_REPRESENTATION ( 'Handle', ( #11957 ), #9978 ) ;
#6224=CARTESIAN_POINT ( 'NONE',  ( -827.8051113588386443, 81.72309053119306554, -154.3319006730158094 ) ) ;
#6225=CARTESIAN_POINT ( 'NONE',  ( -953.2897746444517679, 79.65961628290871488, -95.06748246948048120 ) ) ;
#6236=CARTESIAN_POINT ( 'NONE',  ( -904.2101318205999405, 125.2895275102983419, -124.6807709998041531 ) ) ;
#6238=DIRECTION ( 'NONE',  ( 1.000000000000000000, -1.262554838833776231E-16, 0.000000000000000000 ) ) ;
#6246=CARTESIAN_POINT ( 'NONE',  ( -1038.158164256572263, 71.32123499372137587, -154.2940595301283224 ) ) ;
#6247=CARTESIAN_POINT ( 'NONE',  ( -821.7324155770304515, 74.13196894618619126, -143.0682369473090603 ) ) ;
#6251=CARTESIAN_POINT ( 'NONE',  ( -828.1700845326885201, 76.17242124353187194, -94.68660788644223203 ) ) ;
#6255=CARTESIAN_POINT ( 'NONE',  ( -853.7969483066773364, 45.36294356226267865, -149.7857175106635168 ) ) ;
#6266=CARTESIAN_POINT ( 'NONE',  ( -957.2086549536783195, 47.65337959301152893, -126.6442663926291345 ) ) ;
#6268=AXIS2_PLACEMENT_3D ( 'NONE', #3785, #2804, #1883 ) ;
#6269=CARTESIAN_POINT ( 'NONE',  ( -819.0864923327435463, 80.29251723649532835, -154.5226158375324985 ) ) ;
#6270=CARTESIAN_POINT ( 'NONE',  ( -1031.956718292106189, 74.21439239895558160, -95.06748246948035330 ) ) ;
#6279=CARTESIAN_POINT ( 'NONE',  ( -827.5986411883342271, 81.97471746463595821, -154.3043682292991718 ) ) ;
#6280=CARTESIAN_POINT ( 'NONE',  ( -1038.028607166439997, 78.75533988487829617, -94.48732055948607922 ) ) ;
#6283=AXIS2_PLACEMENT_3D ( 'NONE', #11239, #6528, #10298 ) ;
#6292=CARTESIAN_POINT ( 'NONE',  ( -1021.743962174751232, 119.2557508373789403, -122.7172756069789585 ) ) ;
#6293=DIRECTION ( 'NONE',  ( -1.000000000000000000, 1.262554838833776231E-16, 0.000000000000000000 ) ) ;
#6302=CARTESIAN_POINT ( 'NONE',  ( -821.5848584200534788, 74.20299736547815428, -143.0985335409777690 ) ) ;
#6306=CARTESIAN_POINT ( 'NONE',  ( -974.9912860506709649, 88.33816101283774458, -154.2940595301278108 ) ) ;
#6313=CARTESIAN_POINT ( 'NONE',  ( -817.7441816825903516, 35.12288937987674586, -141.4553492942758908 ) ) ;
#6326=DIRECTION ( 'NONE',  ( 0.000000000000000000, 5.522905491341382306E-16, 1.000000000000000000 ) ) ;
#6328=CARTESIAN_POINT ( 'NONE',  ( -1031.632959140997855, 88.47632675500361188, -95.06748246948018277 ) ) ;
#6334=EDGE_LOOP ( 'NONE', ( #2248, #6155 ) ) ;
#6336=CARTESIAN_POINT ( 'NONE',  ( -1020.430183747026263, 74.13649791779302234, -96.78565065507955012 ) ) ;
#6349=CARTESIAN_POINT ( 'NONE',  ( -1065.000000000008868, 109.8950841424299512, -113.1262384684097526 ) ) ;
#6360=CARTESIAN_POINT ( 'NONE',  ( -1019.365209469141632, 93.24061105504456748, -154.2940595301284361 ) ) ;
#6372=CARTESIAN_POINT ( 'NONE',  ( -1015.825132819589953, 80.44428838836770979, -154.2940595301284645 ) ) ;
#6391=CARTESIAN_POINT ( 'NONE',  ( -818.8285638327253082, 79.00501984256794685, -154.6082502017302147 ) ) ;
#6392=CARTESIAN_POINT ( 'NONE',  ( -853.5732225365160275, 62.99598188221410311, -95.06748246948041015 ) ) ;
#6403=CARTESIAN_POINT ( 'NONE',  ( -1027.375436305349467, 71.63039521860197567, -96.78565065507956433 ) ) ;
#6417=CARTESIAN_POINT ( 'NONE',  ( -1017.840614713424657, 119.3387310954205986, -118.7903414690676556 ) ) ;
#6429=CARTESIAN_POINT ( 'NONE',  ( -1046.676250823071769, 92.10743237175765330, -152.5758913445291967 ) ) ;
#6433=CARTESIAN_POINT ( 'NONE',  ( -1015.209561144950953, 93.46821065761417913, -154.2940595301282656 ) ) ;
#6439=CARTESIAN_POINT ( 'NONE',  ( -953.2897746444480163, 79.65961628290892804, -154.2940595301281519 ) ) ;
#6455=CARTESIAN_POINT ( 'NONE',  ( -1026.284439350007460, 91.37828661775220951, -95.06748246948018277 ) ) ;
#6458=CARTESIAN_POINT ( 'NONE',  ( -1014.132585063772808, 52.13780504951625261, -126.6442663926290777 ) ) ;
#6459=CARTESIAN_POINT ( 'NONE',  ( -820.9141234758983501, 82.74039896267174754, -144.6672699209830739 ) ) ;
#6467=CARTESIAN_POINT ( 'NONE',  ( -1048.040919118596321, 50.77060569800394063, -103.3307627799636919 ) ) ;
#6470=CYLINDRICAL_SURFACE ( 'NONE', #4989, 5.000000000000115463 ) ;
#6481=CARTESIAN_POINT ( 'NONE',  ( -1011.051362836439694, 118.1813008219151868, -113.1262384684097952 ) ) ;
#6491=CARTESIAN_POINT ( 'NONE',  ( -1018.692594135740137, 105.1726068785159214, -149.7857175106633747 ) ) ;
#6493=FACE_BOUND ( 'NONE', #11863, .T. ) ;
#6494=CARTESIAN_POINT ( 'NONE',  ( -1019.365209469141632, 93.24061105504456748, -154.2940595301284361 ) ) ;
#6500=CARTESIAN_POINT ( 'NONE',  ( -1026.651933061287082, 84.71212313386841686, -154.8742214401230228 ) ) ;
#6507=CARTESIAN_POINT ( 'NONE',  ( -1062.810894920117335, 52.92335929224806534, -141.4553492942755781 ) ) ;
#6520=CARTESIAN_POINT ( 'NONE',  ( -1065.000000000009095, 65.22545431197600863, -99.57582448894517313 ) ) ;
#6527=CARTESIAN_POINT ( 'NONE',  ( -1028.007066121602975, 60.50166182213163069, -103.3307627799636350 ) ) ;
#6528=DIRECTION ( 'NONE',  ( -1.000000000000000000, 1.262554838833776231E-16, 0.000000000000000000 ) ) ;
#6540=CARTESIAN_POINT ( 'NONE',  ( -1022.396981161626059, 109.5926079579672319, -103.3307627799638482 ) ) ;
#6550=CARTESIAN_POINT ( 'NONE',  ( -821.0802431487052218, 81.36881375820613016, -154.2940595301280382 ) ) ;
#6558=LINE ( 'NONE', #2727, #2667 ) ;
#6563=CARTESIAN_POINT ( 'NONE',  ( -903.0443340174343803, 90.92133391050434454, -154.8742214401225112 ) ) ;
#6571=CARTESIAN_POINT ( 'NONE',  ( -1028.259718048100012, 56.21337363619606720, -141.4553492942759476 ) ) ;
#6582=CARTESIAN_POINT ( 'NONE',  ( -1025.323167507843664, 62.35287014669171413, -103.3307627799636350 ) ) ;
#6583=CARTESIAN_POINT ( 'NONE',  ( -820.0579670039606981, 81.97422455664163010, -104.6794498541746208 ) ) ;
#6589=CARTESIAN_POINT ( 'NONE',  ( -1016.863910020555409, 59.13213530333446499, -107.9061927053325576 ) ) ;
#6590=AXIS2_PLACEMENT_3D ( 'NONE', #10560, #2962, #9513 ) ;
#6601=CARTESIAN_POINT ( 'NONE',  ( -852.8684863605087685, 118.0406360202081970, -136.2353035311977862 ) ) ;
#6603=CARTESIAN_POINT ( 'NONE',  ( -974.2138504089111848, 120.9496320545084984, -113.1262384684093547 ) ) ;
#6609=CARTESIAN_POINT ( 'NONE',  ( -1045.864486809339951, 115.5688325305733741, -122.7172756069790438 ) ) ;
#6611=CARTESIAN_POINT ( 'NONE',  ( -904.2101318205999405, 125.2895275102983419, -124.6807709998041531 ) ) ;
#6614=CARTESIAN_POINT ( 'NONE',  ( -1031.197907781699314, 107.2697845108579173, -146.0307792196445291 ) ) ;
#6622=CARTESIAN_POINT ( 'NONE',  ( -975.1903095749692056, 79.73237568579439483, -154.8742214401228523 ) ) ;
#6629=CARTESIAN_POINT ( 'NONE',  ( -824.9897882054075353, 73.80822682503037413, -106.4353286633425029 ) ) ;
#6634=ADVANCED_FACE ( 'NONE', ( #6493, #9210 ), #10269, .F. ) ;
#6637=PRODUCT ( 'Handle', 'Handle', '', ( #3989 ) ) ;
#6641=CARTESIAN_POINT ( 'NONE',  ( -927.9936929689729368, 74.21188826700399943, -99.57582448894522997 ) ) ;
#6650=CARTESIAN_POINT ( 'NONE',  ( -1013.392840968506675, 67.31954129910425877, -99.57582448894551419 ) ) ;
#6656=CARTESIAN_POINT ( 'NONE',  ( -974.2138504089111848, 120.9496320545084984, -113.1262384684093547 ) ) ;
#6662=CARTESIAN_POINT ( 'NONE',  ( -1025.296800000965050, 108.9225844456047696, -103.3307627799635782 ) ) ;
#6663=CARTESIAN_POINT ( 'NONE',  ( -926.5908784743301112, 123.4113341959662762, -136.2353035311976441 ) ) ;
#6668=CARTESIAN_POINT ( 'NONE',  ( -1017.810720698610226, 119.7719591276204625, -122.7172756069789017 ) ) ;
#6673=CARTESIAN_POINT ( 'NONE',  ( -853.0139081111152564, 107.1087209265616735, -146.0307792196445291 ) ) ;
#6684=CARTESIAN_POINT ( 'NONE',  ( -828.3216978517767757, 80.87401637003937083, -144.6495766896184421 ) ) ;
#6685=CARTESIAN_POINT ( 'NONE',  ( -821.5852935318529262, 74.19369191907395589, -106.2666214282633490 ) ) ;
#6686=CARTESIAN_POINT ( 'NONE',  ( -954.0832773815118344, 60.15510303592687080, -146.0307792196447565 ) ) ;
#6694=CARTESIAN_POINT ( 'NONE',  ( -1017.027421246632343, 56.01181809833700243, -136.2353035311990368 ) ) ;
#6699=CARTESIAN_POINT ( 'NONE',  ( -928.1401715908999677, 69.16346707076998257, -103.3307627799636919 ) ) ;
#6701=CARTESIAN_POINT ( 'NONE',  ( -819.0811117622716893, 80.27710935352847343, -104.7528066153024042 ) ) ;
#6709=CARTESIAN_POINT ( 'NONE',  ( -902.4158961391592584, 71.79205886009090420, -99.57582448894511629 ) ) ;
#6720=CARTESIAN_POINT ( 'NONE',  ( -822.7482738817717518, 104.4536172844453858, -103.3307627799637203 ) ) ;
#6723=CARTESIAN_POINT ( 'NONE',  ( -1030.931480980269043, 117.9615145441170654, -122.7172756069790722 ) ) ;
#6727=CARTESIAN_POINT ( 'NONE',  ( -992.1517139731079169, 115.6613254010897123, -141.4553492942762318 ) ) ;
#6735=CARTESIAN_POINT ( 'NONE',  ( -1060.958858734060186, 107.4804882715809526, -141.4553492942761750 ) ) ;
#6741=CARTESIAN_POINT ( 'NONE',  ( -1065.000000000001364, 65.22545431197576704, -149.7857175106635168 ) ) ;
#6754=CARTESIAN_POINT ( 'NONE',  ( -975.9242088207895449, 48.36955882740807766, -103.3307627799632513 ) ) ;
#6755=CARTESIAN_POINT ( 'NONE',  ( -828.8285638327245124, 78.83536470145031672, -104.9320557148181479 ) ) ;
#6756=CARTESIAN_POINT ( 'NONE',  ( -928.4218612484578443, 59.99049470396625594, -130.5712005305400965 ) ) ;
#6759=CARTESIAN_POINT ( 'NONE',  ( -827.5977362841322247, 75.37243826020210236, -154.6813451849070304 ) ) ;
#6764=CARTESIAN_POINT ( 'NONE',  ( -1032.589060384100776, 47.36392975189028931, -113.1262384684095537 ) ) ;
#6771=CARTESIAN_POINT ( 'NONE',  ( -991.8293279264787543, 119.7328159579555091, -113.1262384684096673 ) ) ;
#6779=CARTESIAN_POINT ( 'NONE',  ( -1031.329434936836833, 101.6864263019767378, -99.57582448894520155 ) ) ;
#6789=CARTESIAN_POINT ( 'NONE',  ( -1037.461794897090840, 110.6138330393710731, -141.4553492942763171 ) ) ;
#6798=CARTESIAN_POINT ( 'NONE',  ( -1018.401127491266152, 110.2021201405462136, -146.0307792196445860 ) ) ;
#6807=CARTESIAN_POINT ( 'NONE',  ( -1047.626240907250804, 63.12837257276900260, -152.5758913445295093 ) ) ;
#6814=CIRCLE ( 'NONE', #1485, 20.00000000000017053 ) ;
#6821=CARTESIAN_POINT ( 'NONE',  ( -795.0000000000020464, 54.10491585757070965, -113.1262384684093121 ) ) ;
#6823=CARTESIAN_POINT ( 'NONE',  ( -822.0624079427843753, 83.35484814232698625, -104.7266156443422176 ) ) ;
#6824=CARTESIAN_POINT ( 'NONE',  ( -1032.589060384111690, 47.36392975189053800, -136.2353035311989231 ) ) ;
#6831=CARTESIAN_POINT ( 'NONE',  ( -1028.611899521406713, 50.57492120214472919, -122.7172756069792428 ) ) ;
#6837=CARTESIAN_POINT ( 'NONE',  ( -823.1749794181283733, 110.1592441374100844, -107.9061927053325292 ) ) ;
#6846=CARTESIAN_POINT ( 'NONE',  ( -903.6727718956999524, 110.0506089609176712, -99.57582448894470417 ) ) ;
#6849=CARTESIAN_POINT ( 'NONE',  ( -795.0000000000021600, 107.1049510380564129, -141.4553492942762318 ) ) ;
#6851=CARTESIAN_POINT ( 'NONE',  ( -1065.000000000006594, 112.0000000000007105, -124.6807709998041531 ) ) ;
#6858=CARTESIAN_POINT ( 'NONE',  ( -1011.211222789229396, 114.9684118750914621, -141.4553492942763455 ) ) ;
#6862=EDGE_LOOP ( 'NONE', ( #10878, #9601 ) ) ;
#6863=CARTESIAN_POINT ( 'NONE',  ( -951.4198147059590838, 125.0824040815807194, -126.6442663926291345 ) ) ;
#6871=CARTESIAN_POINT ( 'NONE',  ( -817.7441816825903516, 35.12288937987674586, -141.4553492942758908 ) ) ;
#6872=CARTESIAN_POINT ( 'NONE',  ( -818.8285638327238303, 78.67432280806571043, -144.4023295390032899 ) ) ;
#6881=CARTESIAN_POINT ( 'NONE',  ( -1021.607260580486013, 54.24386729702176524, -118.7903414690683661 ) ) ;
#6883=CARTESIAN_POINT ( 'NONE',  ( -997.7839878466141954, 40.27522178589210711, -136.2353035311988378 ) ) ;
#6892=CARTESIAN_POINT ( 'NONE',  ( -1028.581275045472694, 51.02622020309998163, -118.7903414690682240 ) ) ;
#6895=CARTESIAN_POINT ( 'NONE',  ( -822.7482738817717518, 104.4536172844453858, -103.3307627799637203 ) ) ;
#6902=CARTESIAN_POINT ( 'NONE',  ( -1019.017691546883157, 99.44610047464911418, -96.78565065507929432 ) ) ;
#6905=CARTESIAN_POINT ( 'NONE',  ( -1045.884592419587534, 115.0579440276406871, -130.5712005305406365 ) ) ;
#6906=CARTESIAN_POINT ( 'NONE',  ( -926.5289067496701136, 125.3297071905304989, -130.5712005305407786 ) ) ;
#6930=CARTESIAN_POINT ( 'NONE',  ( -819.4847856676407218, 76.17713329584785242, -105.5450962460541149 ) ) ;
#6931=CARTESIAN_POINT ( 'NONE',  ( -1020.755281158171670, 68.40999151392655619, -149.7857175106638010 ) ) ;
#6936=EDGE_LOOP ( 'NONE', ( #9755, #10032 ) ) ;
#6940=CARTESIAN_POINT ( 'NONE',  ( -957.1839320239914741, 48.17551948191501765, -118.7903414690682951 ) ) ;
#6943=CARTESIAN_POINT ( 'NONE',  ( -957.0819499390250940, 50.45265437475578807, -136.2353035311988663 ) ) ;
#6952=CARTESIAN_POINT ( 'NONE',  ( -1048.438004920982848, 39.66697241395321782, -126.6442663926296603 ) ) ;
#6956=CARTESIAN_POINT ( 'NONE',  ( -1055.469533842434430, 91.91071092603658599, -96.78565065507918064 ) ) ;
#6962=CARTESIAN_POINT ( 'NONE',  ( -1025.595388641369482, 103.7168792382126128, -99.57582448894517313 ) ) ;
#6963=CARTESIAN_POINT ( 'NONE',  ( -1021.777026427250121, 118.8177985574659346, -130.5712005305405228 ) ) ;
#6964=CARTESIAN_POINT ( 'NONE',  ( -1024.691966601151762, 118.8493250655917564, -126.6442663926291061 ) ) ;
#6972=CARTESIAN_POINT ( 'NONE',  ( -1014.132585063772581, 52.13780504951625261, -124.6807709998041531 ) ) ;
#6977=CARTESIAN_POINT ( 'NONE',  ( -974.1288507787422759, 124.2142274477005657, -124.6807709998040110 ) ) ;
#6985=CARTESIAN_POINT ( 'NONE',  ( -1061.884876827093876, 80.20192378191431715, -154.8742214401230797 ) ) ;
#6995=CARTESIAN_POINT ( 'NONE',  ( -1057.521967982373098, 48.25222617153974625, -141.4553492942758623 ) ) ;
#7000=CARTESIAN_POINT ( 'NONE',  ( -1032.658196452834773, 44.72920460984212809, -122.7172756069792143 ) ) ;
#7005=CARTESIAN_POINT ( 'NONE',  ( -822.2158551983004600, 73.93035145837139055, -154.6498254730319957 ) ) ;
#7009=CARTESIAN_POINT ( 'NONE',  ( -1028.611899521407167, 50.57492120214475761, -126.6442663926292340 ) ) ;
#7012=CARTESIAN_POINT ( 'NONE',  ( -828.8285638327243987, 78.67432280806561096, -104.9592124606052863 ) ) ;
#7015=CARTESIAN_POINT ( 'NONE',  ( -1011.935294340108044, 99.50314415908297860, -96.78565065507922327 ) ) ;
#7021=CARTESIAN_POINT ( 'NONE',  ( -820.5239792770877330, 82.44072200957887731, -154.2973869372356432 ) ) ;
#7022=CARTESIAN_POINT ( 'NONE',  ( -954.7734463792770612, 107.7731650919851205, -99.57582448894495997 ) ) ;
#7024=CARTESIAN_POINT ( 'NONE',  ( -1037.337636019037518, 116.9882293220590270, -126.6442663926289640 ) ) ;
#7027=CARTESIAN_POINT ( 'NONE',  ( -1017.840614713424657, 119.3387310954205986, -118.7903414690676556 ) ) ;
#7034=CARTESIAN_POINT ( 'NONE',  ( -818.9564113685823941, 79.80952029794852365, -94.80345787799255675 ) ) ;
#7049=( NAMED_UNIT ( * ) PLANE_ANGLE_UNIT ( ) SI_UNIT ( $, .RADIAN. ) );
#7052=CARTESIAN_POINT ( 'NONE',  ( -1057.299536696276846, 52.76571712355565325, -146.0307792196449554 ) ) ;
#7058=CARTESIAN_POINT ( 'NONE',  ( -795.0000000000061391, 52.38665522077228331, -118.7903414690680250 ) ) ;
#7064=ADVANCED_BREP_SHAPE_REPRESENTATION ( '', ( #8008, #11957 ), #9978 ) ;
#7071=CARTESIAN_POINT ( 'NONE',  ( -795.0000000000079581, 93.55451860843940892, -96.78565065507920906 ) ) ;
#7083=CARTESIAN_POINT ( 'NONE',  ( -955.6263874535618470, 86.32439835342511003, -94.48732055948597974 ) ) ;
#7085=CLOSED_SHELL ( 'NONE', ( #7655, #1780, #6634, #1634, #4424, #975, #1592, #10297, #9276, #9329, #4579 ) ) ;
#7094=CARTESIAN_POINT ( 'NONE',  ( -901.8785362142588156, 56.55314031071017666, -124.6807709998039968 ) ) ;
#7096=CARTESIAN_POINT ( 'NONE',  ( -819.3351944727438649, 80.89172441788861079, -94.89089580185901696 ) ) ;
#7100=CARTESIAN_POINT ( 'NONE',  ( -954.0441199534440102, 124.9954171138387977, -124.6807709998039115 ) ) ;
#7108=CARTESIAN_POINT ( 'NONE',  ( -1012.828629370413182, 79.69572830938452057, -154.2940595301284361 ) ) ;
#7109=CARTESIAN_POINT ( 'NONE',  ( -828.6674387974398996, 77.37343372931326257, -144.1410586993683012 ) ) ;
#7112=CARTESIAN_POINT ( 'NONE',  ( -827.8046876470999678, 75.62493715853115361, -94.68085105088540843 ) ) ;
#7117=CARTESIAN_POINT ( 'NONE',  ( -953.8433812051875975, 65.95343150956774991, -149.7857175106634315 ) ) ;
#7133=CARTESIAN_POINT ( 'NONE',  ( -1065.000000000005912, 82.00000000000039790, -94.48732055948609343 ) ) ;
#7146=CARTESIAN_POINT ( 'NONE',  ( -820.4595805503671500, 72.64106675864344709, -94.48732055948583763 ) ) ;
#7148=CARTESIAN_POINT ( 'NONE',  ( -1010.922847972424620, 120.6260792194949829, -126.6442663926288503 ) ) ;
#7152=CARTESIAN_POINT ( 'NONE',  ( -1060.846413679908210, 110.5345601522217720, -113.1262384684099374 ) ) ;
#7162=CARTESIAN_POINT ( 'NONE',  ( -954.0688428831313104, 124.4732772249355577, -118.7903414690677693 ) ) ;
#7172=CARTESIAN_POINT ( 'NONE',  ( -823.4903519156995344, 73.67469885889941850, -142.8656372648663080 ) ) ;
#7177=AXIS2_PLACEMENT_3D ( 'NONE', #4979, #279, #4067 ) ;
#7180=CARTESIAN_POINT ( 'NONE',  ( -1028.259718048100012, 56.21337363619606720, -141.4553492942759476 ) ) ;
#7189=ORIENTED_EDGE ( 'NONE', *, *, #7970, .T. ) ;
#7195=EDGE_CURVE ( 'NONE', #5919, #9092, #12224, .T. ) ;
#7197=CARTESIAN_POINT ( 'NONE',  ( -1019.365209469143679, 93.24061105504411273, -95.06748246948018277 ) ) ;
#7205=( LENGTH_UNIT ( ) NAMED_UNIT ( * ) SI_UNIT ( .MILLI., .METRE. ) );
#7208=CARTESIAN_POINT ( 'NONE',  ( -823.1748664167885181, 83.64213179714484170, -154.1150047552051490 ) ) ;
#7210=CARTESIAN_POINT ( 'NONE',  ( -991.5701548301636876, 122.8678427087060214, -124.6807709998040536 ) ) ;
#7211=B_SPLINE_CURVE_WITH_KNOTS ( 'NONE', 3,
 ( #4936, #4194, #7972, #7034, #10804, #2344, #11798, #7096, #3314, #6115, #10859, #9882, #5174, #5230, #9002, #9936, #1472, #4317, #535, #432, #5144, #4164, #4222, #9726, #11770, #8905, #4291, #8974, #7938, #499, #11829, #8000, #10888, #9784, #4109, #9030, #11711, #570, #3286, #3224 ),
 .UNSPECIFIED., .F., .F.,
 ( 4, 2, 2, 2, 2, 2, 2, 2, 2, 2, 2, 2, 2, 2, 2, 2, 2, 2, 2, 4 ),
 ( 0.000000000000000000, 0.0009792129545681763775, 0.001468819431852298393, 0.001958425909136420843, 0.002937638863704576404, 0.003916851818272732398, 0.004896064772840888826, 0.005875277727409044387, 0.006854490681977199081, 0.007833703636545355509, 0.008812916591113511069, 0.009792129545681668365, 0.01028173602296574528, 0.01077134250024982393, 0.01175055545481823276, 0.01272976840938664506, 0.01321937488667085207, 0.01370898136395505736, 0.01468819431852334649, 0.01566740727309163389 ),
 .UNSPECIFIED. ) ;
#7219=CARTESIAN_POINT ( 'NONE',  ( -819.3349937000580212, 76.45728329316879979, -154.6806410948596806 ) ) ;
#7223=CARTESIAN_POINT ( 'NONE',  ( -1045.884592419585942, 115.0579440276405450, -118.7903414690682524 ) ) ;
#7235=CARTESIAN_POINT ( 'NONE',  ( -822.4997677527437645, 73.84243176666275588, -142.9416447491881286 ) ) ;
#7243=CARTESIAN_POINT ( 'NONE',  ( -1025.323167507848893, 62.35287014669186334, -146.0307792196450691 ) ) ;
#7253=ORIENTED_EDGE ( 'NONE', *, *, #3438, .T. ) ;
#7269=CARTESIAN_POINT ( 'NONE',  ( -1024.256845364730452, 79.46673622094698430, -95.06748246948041015 ) ) ;
#7271=FACE_OUTER_BOUND ( 'NONE', #5574, .T. ) ;
#7281=CARTESIAN_POINT ( 'NONE',  ( -819.0908945849121210, 77.06763757931493330, -154.6734934370493306 ) ) ;
#7285=DIRECTION ( 'NONE',  ( -4.236366511936864528E-16, 1.000000000000000000, 5.522905491341393153E-16 ) ) ;
#7286=CARTESIAN_POINT ( 'NONE',  ( -1013.901471336336158, 119.8325901201402814, -118.7903414690677835 ) ) ;
#7296=CARTESIAN_POINT ( 'NONE',  ( -1017.810720698609543, 119.7719591276204625, -124.6807709998040679 ) ) ;
#7299=CARTESIAN_POINT ( 'NONE',  ( -927.1204550305436669, 105.3607176047074745, -152.5758913445291114 ) ) ;
#7303=CARTESIAN_POINT ( 'NONE',  ( -927.1204550305436669, 105.3607176047074745, -152.5758913445291114 ) ) ;
#7308=EDGE_CURVE ( 'NONE', #9092, #4723, #6558, .T. ) ;
#7311=CARTESIAN_POINT ( 'NONE',  ( -1032.113539130925574, 67.34854938887519893, -152.5758913445294240 ) ) ;
#7326=CARTESIAN_POINT ( 'NONE',  ( -952.6992609796628813, 94.45070821374962122, -95.06748246947989855 ) ) ;
#7345=CARTESIAN_POINT ( 'NONE',  ( -1060.846413679908210, 110.5345601522217720, -113.1262384684099374 ) ) ;
#7357=CARTESIAN_POINT ( 'NONE',  ( -1023.078931369431530, 98.73915068298377662, -152.5758913445292535 ) ) ;
#7362=CARTESIAN_POINT ( 'NONE',  ( -853.2189900670995257, 91.12674563889149226, -152.5758913445289693 ) ) ;
#7367=CARTESIAN_POINT ( 'NONE',  ( -819.2376510598713821, 55.50059629688480811, -152.5758913445292535 ) ) ;
#7378=CARTESIAN_POINT ( 'NONE',  ( -818.8285638327251945, 78.67432280806566780, -154.6235849673217899 ) ) ;
#7385=CARTESIAN_POINT ( 'NONE',  ( -819.3361059452977315, 80.89324539545522441, -154.4704897894791031 ) ) ;
#7387=CARTESIAN_POINT ( 'NONE',  ( -1056.743458481016432, 64.45745743522633120, -96.78565065507969223 ) ) ;
#7398=CARTESIAN_POINT ( 'NONE',  ( -975.9242088207895449, 48.36955882740807766, -103.3307627799632513 ) ) ;
#7410=CARTESIAN_POINT ( 'NONE',  ( -1061.104375862967800, 103.3839434440458547, -103.3307627799635924 ) ) ;
#7418=CARTESIAN_POINT ( 'NONE',  ( -1021.743962174751232, 119.2557508373789403, -124.6807709998040110 ) ) ;
#7421=CARTESIAN_POINT ( 'NONE',  ( -1011.935294340112478, 99.50314415908300703, -152.5758913445291967 ) ) ;
#7427=CARTESIAN_POINT ( 'NONE',  ( -1056.106496161729183, 78.18408418063155807, -154.8742214401234776 ) ) ;
#7444=CARTESIAN_POINT ( 'NONE',  ( -795.0000000000022737, 65.22545431197607968, -99.57582448894522997 ) ) ;
#7455=CARTESIAN_POINT ( 'NONE',  ( -1025.323167507843664, 62.35287014669171413, -103.3307627799636350 ) ) ;
#7458=DIRECTION ( 'NONE',  ( -1.000000000000000000, -4.236366511936864528E-16, -3.037002292462560327E-31 ) ) ;
#7472=CARTESIAN_POINT ( 'NONE',  ( -1054.913455627178109, 103.6024512377076263, -103.3307627799635640 ) ) ;
#7482=CARTESIAN_POINT ( 'NONE',  ( -975.1903095749692056, 79.73237568579439483, -154.8742214401228523 ) ) ;
#7492=CARTESIAN_POINT ( 'NONE',  ( -1031.794838716557251, 81.34535957697963227, -154.8742214401231649 ) ) ;
#7496=CARTESIAN_POINT ( 'NONE',  ( -828.6712641482290564, 79.96111424986135319, -144.5792126457448603 ) ) ;
#7497=CARTESIAN_POINT ( 'NONE',  ( -826.0807747705229076, 74.19805998537532332, -106.2647609865424556 ) ) ;
#7509=CARTESIAN_POINT ( 'NONE',  ( -1057.521967982379238, 48.25222617154000204, -107.9061927053324723 ) ) ;
#7510=CARTESIAN_POINT ( 'NONE',  ( -818.8285638327240576, 78.67432280806558254, -104.9592124606052295 ) ) ;
#7512=CARTESIAN_POINT ( 'NONE',  ( -795.0000000000036380, 52.00000000000027711, -126.6442663926292624 ) ) ;
#7518=CARTESIAN_POINT ( 'NONE',  ( -1028.259718048105469, 56.21337363619640115, -107.9061927053325434 ) ) ;
#7519=FACE_OUTER_BOUND ( 'NONE', #12026, .T. ) ;
#7521=CARTESIAN_POINT ( 'NONE',  ( -823.8285638327243987, 78.67432280806571043, -264.6807709998050200 ) ) ;
#7525=EDGE_CURVE ( 'NONE', #4723, #11269, #5732, .T. ) ;
#7531=CARTESIAN_POINT ( 'NONE',  ( -951.5459139781289650, 122.3346817490815681, -113.1262384684093263 ) ) ;
#7536=CARTESIAN_POINT ( 'NONE',  ( -1060.756016675587944, 112.8516620848305934, -122.7172756069790864 ) ) ;
#7541=CARTESIAN_POINT ( 'NONE',  ( -795.0000000000080718, 93.55451860843929524, -152.5758913445291398 ) ) ;
#7548=CARTESIAN_POINT ( 'NONE',  ( -956.2104666674752025, 71.56905446038098262, -152.5758913445294809 ) ) ;
#7555=CARTESIAN_POINT ( 'NONE',  ( -825.4664863774346486, 73.94730815836283000, -106.3734765325343830 ) ) ;
#7566=CARTESIAN_POINT ( 'NONE',  ( -853.7969483066802923, 45.36294356226295577, -99.57582448894520155 ) ) ;
#7567=CARTESIAN_POINT ( 'NONE',  ( -828.7892213480641885, 79.32116703283894310, -104.8603099499567861 ) ) ;
#7568=CARTESIAN_POINT ( 'NONE',  ( -1028.581275045468146, 51.02622020309988216, -130.5712005305406080 ) ) ;
#7575=CARTESIAN_POINT ( 'NONE',  ( -928.2641150402301946, 65.00826535581501275, -107.9061927053325576 ) ) ;
#7590=CARTESIAN_POINT ( 'NONE',  ( -1054.691024341069351, 108.1159421897237110, -107.9061927053325149 ) ) ;
#7593=CARTESIAN_POINT ( 'NONE',  ( -904.0006525278439540, 119.6095687608908378, -141.4553492942759760 ) ) ;
#7597=CARTESIAN_POINT ( 'NONE',  ( -1017.810720698609543, 119.7719591276204625, -124.6807709998040679 ) ) ;
#7602=CARTESIAN_POINT ( 'NONE',  ( -1018.401127491266152, 110.2021201405462136, -146.0307792196445860 ) ) ;
#7619=CARTESIAN_POINT ( 'NONE',  ( -818.8285638327240576, 78.67432280806558254, -104.9592124606052295 ) ) ;
#7620=CARTESIAN_POINT ( 'NONE',  ( -1016.402231264567945, 68.39482517277122042, -149.7857175106636589 ) ) ;
#7627=CARTESIAN_POINT ( 'NONE',  ( -1057.693846703458348, 44.87596864925374973, -136.2353035311986957 ) ) ;
#7630=CARTESIAN_POINT ( 'NONE',  ( -1032.391769651399727, 55.42093464310126905, -103.3307627799637487 ) ) ;
#7631=DIRECTION ( 'NONE',  ( -1.000000000000000000, -4.236366511936864528E-16, -3.037002292462560327E-31 ) ) ;
#7632=CARTESIAN_POINT ( 'NONE',  ( -954.5692209181586350, 49.02792041507773746, -122.7172756069790580 ) ) ;
#7640=CARTESIAN_POINT ( 'NONE',  ( -1048.206790403141440, 45.99070412075073477, -107.9061927053325007 ) ) ;
#7644=CARTESIAN_POINT ( 'NONE',  ( -1031.086615573502741, 111.8776252365149730, -107.9061927053324723 ) ) ;
#7651=CARTESIAN_POINT ( 'NONE',  ( -903.8503739047830550, 115.2915043052427535, -103.3307627799633082 ) ) ;
#7653=CARTESIAN_POINT ( 'NONE',  ( -1010.947924043452645, 120.1731093567702828, -130.5712005305404375 ) ) ;
#7655=ADVANCED_FACE ( 'NONE', ( #8928 ), #11951, .F. ) ;
#7662=CARTESIAN_POINT ( 'NONE',  ( -903.8503739047791896, 115.2915043052427251, -146.0307792196441881 ) ) ;
#7669=CARTESIAN_POINT ( 'NONE',  ( -822.7482738817701602, 104.4536172844453148, -146.0307792196443017 ) ) ;
#7677=CARTESIAN_POINT ( 'NONE',  ( -820.5035528205731907, 74.92619343081619832, -105.9719278460594580 ) ) ;
#7679=CARTESIAN_POINT ( 'NONE',  ( -1038.506348936321501, 51.71309463382193883, -146.0307792196451260 ) ) ;
#7689=CARTESIAN_POINT ( 'NONE',  ( -996.0013826475885708, 63.70094029248571132, -96.78565065507963538 ) ) ;
#7690=CARTESIAN_POINT ( 'NONE',  ( -828.6703486388537385, 79.96407734986419769, -104.7820573548429195 ) ) ;
#7691=CARTESIAN_POINT ( 'NONE',  ( -954.5446161821218993, 49.54000128949421367, -130.5712005305404091 ) ) ;
#7694=CARTESIAN_POINT ( 'NONE',  ( -819.0830098008030973, 80.28235241365214847, -144.6091609974198207 ) ) ;
#7696=CARTESIAN_POINT ( 'NONE',  ( -828.6683600116994057, 77.37701618531993120, -154.6440356896530659 ) ) ;
#7701=CARTESIAN_POINT ( 'NONE',  ( -1065.000000000006594, 52.38665522077229042, -118.7903414690683945 ) ) ;
#7702=CARTESIAN_POINT ( 'NONE',  ( -1065.000000000006594, 112.0000000000007105, -124.6807709998041531 ) ) ;
#7707=LINE ( 'NONE', #3939, #8933 ) ;
#7709=CARTESIAN_POINT ( 'NONE',  ( -795.0000000000070486, 103.3499740386316859, -103.3307627799634218 ) ) ;
#7710=CARTESIAN_POINT ( 'NONE',  ( -1054.407929976944160, 113.5897173251037628, -130.5712005305405228 ) ) ;
#7712=CARTESIAN_POINT ( 'NONE',  ( -823.7697810748812799, 117.7733807739867871, -124.6807709998041531 ) ) ;
#7717=CARTESIAN_POINT ( 'NONE',  ( -1060.846413679901389, 110.5345601522218146, -136.2353035311979852 ) ) ;
#7725=CARTESIAN_POINT ( 'NONE',  ( -952.1456544189259148, 108.1568929870910836, -149.7857175106632042 ) ) ;
#7734=CARTESIAN_POINT ( 'NONE',  ( -853.7969483066773364, 45.36294356226267865, -149.7857175106635168 ) ) ;
#7741=CARTESIAN_POINT ( 'NONE',  ( -1021.607260580477828, 54.24386729702167997, -130.5712005305404659 ) ) ;
#7748=CARTESIAN_POINT ( 'NONE',  ( -853.9759289228104535, 31.63339360934237021, -107.9061927053328986 ) ) ;
#7749=CARTESIAN_POINT ( 'NONE',  ( -828.1711263241255665, 81.17408148015046265, -104.6959820179053935 ) ) ;
#7751=CARTESIAN_POINT ( 'NONE',  ( -795.0000000000020464, 52.38665522077208436, -130.5712005305402670 ) ) ;
#7753=CARTESIAN_POINT ( 'NONE',  ( -819.4849966174467681, 81.17290644373839825, -144.6655594550755382 ) ) ;
#7760=CARTESIAN_POINT ( 'NONE',  ( -1038.719578313838610, 40.52245044769760085, -122.7172756069793707 ) ) ;
#7764=EDGE_CURVE ( 'NONE', #8579, #10282, #6814, .T. ) ;
#7772=CARTESIAN_POINT ( 'NONE',  ( -1046.909978542194949, 84.99913997988220160, -95.06748246948046699 ) ) ;
#7774=LINE ( 'NONE', #7841, #4908 ) ;
#7778=CARTESIAN_POINT ( 'NONE',  ( -904.2101318206010774, 125.2895275102983419, -122.7172756069790580 ) ) ;
#7783=CARTESIAN_POINT ( 'NONE',  ( -1024.848917040341576, 116.4131098345822437, -136.2353035311980420 ) ) ;
#7788=CARTESIAN_POINT ( 'NONE',  ( -974.1288507787421622, 124.2142274477007078, -126.6442663926288787 ) ) ;
#7792=CARTESIAN_POINT ( 'NONE',  ( -1025.595388641371756, 103.7168792382127975, -149.7857175106636021 ) ) ;
#7802=CARTESIAN_POINT ( 'NONE',  ( -928.2641150402240555, 65.00826535581498433, -141.4553492942759476 ) ) ;
#7813=CARTESIAN_POINT ( 'NONE',  ( -1013.844210246976672, 57.79547239392030633, -107.9061927053327423 ) ) ;
#7820=CARTESIAN_POINT ( 'NONE',  ( -821.6140151324020735, 74.17967406092559202, -154.6554517456385440 ) ) ;
#7824=CARTESIAN_POINT ( 'NONE',  ( -1014.132585063772353, 52.13780504951625261, -122.7172756069792428 ) ) ;
#7828=CARTESIAN_POINT ( 'NONE',  ( -974.4564103291414767, 111.0951925441806480, -103.3307627799632371 ) ) ;
#7836=CARTESIAN_POINT ( 'NONE',  ( -822.2439855206088168, 97.57287547056382948, -99.57582448894494576 ) ) ;
#7839=CARTESIAN_POINT ( 'NONE',  ( -852.8274699693135972, 120.9962006285028906, -130.5712005305406933 ) ) ;
#7840=CARTESIAN_POINT ( 'NONE',  ( -1065.000000000002501, 109.8950841424301359, -136.2353035311980136 ) ) ;
#7841=CARTESIAN_POINT ( 'NONE',  ( -955.0000000000038654, 62.00000000000019185, -124.6807709998041815 ) ) ;
#7844=CARTESIAN_POINT ( 'NONE',  ( -951.4444194419894529, 124.5703232071642503, -118.7903414690678829 ) ) ;
#7849=CARTESIAN_POINT ( 'NONE',  ( -951.9057582426059980, 113.9552214607316216, -146.0307792196438754 ) ) ;
#7857=CARTESIAN_POINT ( 'NONE',  ( -1014.170783943998003, 114.7803637426474808, -141.4553492942763171 ) ) ;
#7865=CARTESIAN_POINT ( 'NONE',  ( -853.8938961404190877, 37.86297855175782701, -146.0307792196449554 ) ) ;
#7870=CARTESIAN_POINT ( 'NONE',  ( -821.6148272622868944, 74.17911137529775090, -94.70610353401345094 ) ) ;
#7873=CARTESIAN_POINT ( 'NONE',  ( -1028.454949082223038, 53.01113643315406421, -136.2353035311987810 ) ) ;
#7877=CARTESIAN_POINT ( 'NONE',  ( -1028.581275045472694, 51.02622020309998163, -118.7903414690682240 ) ) ;
#7879=EDGE_LOOP ( 'NONE', ( #2395, #2313, #7887, #10905 ) ) ;
#7887=ORIENTED_EDGE ( 'NONE', *, *, #2424, .T. ) ;
#7888=CARTESIAN_POINT ( 'NONE',  ( -1017.158871447982051, 53.64146012065780411, -122.7172756069791717 ) ) ;
#7895=CARTESIAN_POINT ( 'NONE',  ( -1055.176328965296989, 98.13059730676610570, -99.57582448894517313 ) ) ;
#7901=CARTESIAN_POINT ( 'NONE',  ( -927.2951026182247460, 99.13268410970638911, -95.06748246948001224 ) ) ;
#7903=CARTESIAN_POINT ( 'NONE',  ( -1037.348432443219735, 116.4729352038311987, -130.5712005305406080 ) ) ;
#7904=CARTESIAN_POINT ( 'NONE',  ( -1030.931480980266770, 117.9615145441171933, -126.6442663926290777 ) ) ;
#7907=CARTESIAN_POINT ( 'NONE',  ( -974.1454360724308117, 123.6012932931490127, -118.7903414690677835 ) ) ;
#7917=CARTESIAN_POINT ( 'NONE',  ( -795.0000000000035243, 112.0000000000008953, -126.6442663926293477 ) ) ;
#7919=CARTESIAN_POINT ( 'NONE',  ( -1014.382386707152364, 110.5980896718283759, -146.0307792196445291 ) ) ;
#7925=CARTESIAN_POINT ( 'NONE',  ( -819.8405841167685821, 75.64117232352727171, -143.6450765909193876 ) ) ;
#7930=CARTESIAN_POINT ( 'NONE',  ( -997.4616017999776432, 44.34671234275830187, -141.4553492942759476 ) ) ;
#7936=CARTESIAN_POINT ( 'NONE',  ( -1025.976186494711783, 52.68972726728017619, -122.7172756069792428 ) ) ;
#7938=CARTESIAN_POINT ( 'NONE',  ( -827.1323880180814285, 82.44176594610610209, -95.11041087168378283 ) ) ;
#7941=CARTESIAN_POINT ( 'NONE',  ( -828.7959811946850550, 78.01751516534540087, -154.6175107292156952 ) ) ;
#7944=CARTESIAN_POINT ( 'NONE',  ( -901.8785362142587019, 56.55314031071017666, -122.7172756069789017 ) ) ;
#7949=CARTESIAN_POINT ( 'NONE',  ( -1019.017691546883157, 99.44610047464911418, -96.78565065507929432 ) ) ;
#7955=DIRECTION ( 'NONE',  ( 1.000000000000000000, 0.000000000000000000, 0.000000000000000000 ) ) ;
#7959=CARTESIAN_POINT ( 'NONE',  ( -1056.106496161727136, 78.18408418063160070, -94.48732055948630659 ) ) ;
#7961=CARTESIAN_POINT ( 'NONE',  ( -904.2101318206000542, 125.2895275102983419, -126.6442663926292340 ) ) ;
#7970=EDGE_CURVE ( 'NONE', #5145, #4637, #341, .T. ) ;
#7972=CARTESIAN_POINT ( 'NONE',  ( -818.8610632455868199, 79.33015038929181628, -94.77164022161367996 ) ) ;
#7983=CARTESIAN_POINT ( 'NONE',  ( -819.1462522098594263, 76.91297450996670193, -144.0236343770281451 ) ) ;
#7990=PRESENTATION_STYLE_ASSIGNMENT (( #9660 ) ) ;
#7993=CARTESIAN_POINT ( 'NONE',  ( -1016.402231264567945, 68.39482517277122042, -149.7857175106636589 ) ) ;
#7999=CARTESIAN_POINT ( 'NONE',  ( -1038.664246639915291, 43.28664065472965206, -113.1262384684093405 ) ) ;
#8000=CARTESIAN_POINT ( 'NONE',  ( -828.0764331662031736, 81.31668519957902674, -94.98799056389854911 ) ) ;
#8008=MANIFOLD_SOLID_BREP ( 'Cut-Extrude4[2]', #7085 ) ;
#8010=CARTESIAN_POINT ( 'NONE',  ( -903.4746773471185861, 104.0883302344921475, -96.78565065507889642 ) ) ;
#8020=CARTESIAN_POINT ( 'NONE',  ( -994.8066578865433485, 80.00401887192406036, -94.48732055948607922 ) ) ;
#8025=CARTESIAN_POINT ( 'NONE',  ( -1010.947924043450712, 120.1731093567701407, -118.7903414690677408 ) ) ;
#8036=CARTESIAN_POINT ( 'NONE',  ( -904.2101318206000542, 125.2895275102983419, -126.6442663926292340 ) ) ;
#8053=CARTESIAN_POINT ( 'NONE',  ( -975.9242088207953429, 48.36955882740826240, -146.0307792196450407 ) ) ;
#8068=CARTESIAN_POINT ( 'NONE',  ( -1037.550865396562358, 105.7975851359348241, -103.3307627799636350 ) ) ;
#8079=CARTESIAN_POINT ( 'NONE',  ( -828.6689926561751918, 79.96979452499502372, -154.4949334293652328 ) ) ;
#8080=CARTESIAN_POINT ( 'NONE',  ( -1065.000000000006139, 76.10956187831460795, -95.06748246948023962 ) ) ;
#8084=CARTESIAN_POINT ( 'NONE',  ( -1045.864486809339269, 115.5688325305735162, -126.6442663926293477 ) ) ;
#8086=CARTESIAN_POINT ( 'NONE',  ( -1065.000000000008868, 109.8950841424299512, -113.1262384684097526 ) ) ;
#8090=CARTESIAN_POINT ( 'NONE',  ( -1063.013736978595261, 47.55218547899809067, -124.6807709998042242 ) ) ;
#8094=CARTESIAN_POINT ( 'NONE',  ( -1060.773655115450993, 112.4236047030758527, -118.7903414690679682 ) ) ;
#8102=CARTESIAN_POINT ( 'NONE',  ( -1056.106496161729183, 78.18408418063155807, -154.8742214401234776 ) ) ;
#8103=CARTESIAN_POINT ( 'NONE',  ( -826.3639150177631336, 74.35254223074741731, -143.1619793993637870 ) ) ;
#8111=CARTESIAN_POINT ( 'NONE',  ( -1021.293373424891683, 59.24127555818969171, -141.4553492942756918 ) ) ;
#8128=CARTESIAN_POINT ( 'NONE',  ( -820.4595805503671500, 72.64106675864344709, -94.48732055948583763 ) ) ;
#8136=CARTESIAN_POINT ( 'NONE',  ( -853.6888141844383426, 53.84495383942796565, -96.78565065507952170 ) ) ;
#8140=CARTESIAN_POINT ( 'NONE',  ( -852.8175266017511831, 121.6828083272127685, -124.6807709998041247 ) ) ;
#8151=CARTESIAN_POINT ( 'NONE',  ( -926.5138833012644000, 125.7648744980332225, -122.7172756069789159 ) ) ;
#8162=CARTESIAN_POINT ( 'NONE',  ( -1031.794838716557251, 81.34535957697963227, -154.8742214401231649 ) ) ;
#8171=CARTESIAN_POINT ( 'NONE',  ( -1032.503061859593117, 50.81309391744441228, -141.4553492942758908 ) ) ;
#8183=CARTESIAN_POINT ( 'NONE',  ( -901.8785362142589292, 56.55314031071017666, -126.6442663926291061 ) ) ;
#8195=CARTESIAN_POINT ( 'NONE',  ( -1020.082665824770629, 80.34198733739781062, -95.06748246948050962 ) ) ;
#8205=CARTESIAN_POINT ( 'NONE',  ( -822.2219070778693322, 83.41200391691957350, -154.1554710663006347 ) ) ;
#8206=CARTESIAN_POINT ( 'NONE',  ( -1013.120138696091999, 73.26074010992823560, -96.78565065507963538 ) ) ;
#8216=CARTESIAN_POINT ( 'NONE',  ( -818.9561402410595292, 77.54029615563084121, -154.6639069421937904 ) ) ;
#8220=CARTESIAN_POINT ( 'NONE',  ( -1065.000000000006594, 112.0000000000007105, -124.6807709998041531 ) ) ;
#8232=CARTESIAN_POINT ( 'NONE',  ( -1037.773541645230580, 93.34895244571352180, -152.5758913445289693 ) ) ;
#8233=CARTESIAN_POINT ( 'NONE',  ( -824.1558762432750882, 73.68222816774749617, -142.8690915370046923 ) ) ;
#8235=DIRECTION ( 'NONE',  ( 1.000000000000000000, -1.262554838833776231E-16, 0.000000000000000000 ) ) ;
#8236=CARTESIAN_POINT ( 'NONE',  ( -955.0423082396526979, 101.0797422464698769, -152.5758913445288272 ) ) ;
#8240=ORIENTED_EDGE ( 'NONE', *, *, #8381, .T. ) ;
#8242=CARTESIAN_POINT ( 'NONE',  ( -996.0013826475917540, 63.70094029248592449, -152.5758913445294240 ) ) ;
#8253=CARTESIAN_POINT ( 'NONE',  ( -823.8285638327243987, 78.67432280806571043, -264.6807709998050200 ) ) ;
#8258=CARTESIAN_POINT ( 'NONE',  ( -953.2897746444517679, 79.65961628290871488, -95.06748246948048120 ) ) ;
#8269=CARTESIAN_POINT ( 'NONE',  ( -825.4463966093486533, 83.41668980410091194, -154.1315809916505088 ) ) ;
#8270=CARTESIAN_POINT ( 'NONE',  ( -927.6556653799030983, 86.18751778479037284, -95.06748246948041015 ) ) ;
#8273=CYLINDRICAL_SURFACE ( 'NONE', #4869, 20.00000000000017053 ) ;
#8287=CARTESIAN_POINT ( 'NONE',  ( -1010.947924043450712, 120.1731093567701407, -118.7903414690677408 ) ) ;
#8299=CARTESIAN_POINT ( 'NONE',  ( -1055.469533842436022, 91.91071092603651493, -152.5758913445291398 ) ) ;
#8300=CARTESIAN_POINT ( 'NONE',  ( -823.1581254408829409, 73.70809864670252409, -142.8810402703306863 ) ) ;
#8303=CARTESIAN_POINT ( 'NONE',  ( -1026.284439350006778, 91.37828661775253636, -154.2940595301281803 ) ) ;
#8309=CARTESIAN_POINT ( 'NONE',  ( -1027.019426772554198, 78.04595964998465263, -154.2940595301285782 ) ) ;
#8316=CARTESIAN_POINT ( 'NONE',  ( -795.0000000000039790, 54.10491585757074517, -136.2353035311982410 ) ) ;
#8324=CARTESIAN_POINT ( 'NONE',  ( -1065.000000000001364, 70.44548139156162847, -96.78565065507940801 ) ) ;
#8327=CARTESIAN_POINT ( 'NONE',  ( -1017.158871447983074, 53.64146012065780411, -126.6442663926291061 ) ) ;
#8328=CARTESIAN_POINT ( 'NONE',  ( -820.5266942580660725, 82.43260598963610164, -144.6763645173222130 ) ) ;
#8334=CARTESIAN_POINT ( 'NONE',  ( -996.5513353153756952, 56.29506814688433280, -99.57582448894517313 ) ) ;
#8357=CARTESIAN_POINT ( 'NONE',  ( -795.0000000000043201, 102.0000000000005684, -124.6807709998040963 ) ) ;
#8359=CARTESIAN_POINT ( 'NONE',  ( -927.2951026182241776, 99.13268410970675859, -154.2940595301278961 ) ) ;
#8370=CARTESIAN_POINT ( 'NONE',  ( -794.9999999999992042, 76.10956187831466480, -154.2940595301278393 ) ) ;
#8376=CARTESIAN_POINT ( 'NONE',  ( -827.8143761345677376, 75.63828352384309994, -105.7174308425206419 ) ) ;
#8377=CARTESIAN_POINT ( 'NONE',  ( -954.4431216459919369, 51.77564274757662588, -136.2353035311985820 ) ) ;
#8381=EDGE_CURVE ( 'NONE', #10282, #1185, #11120, .T. ) ;
#8402=CARTESIAN_POINT ( 'NONE',  ( -818.1708872189576596, 40.82851623284144438, -103.3307627799635640 ) ) ;
#8405=DIRECTION ( 'NONE',  ( 1.000000000000000000, -1.262554838833776231E-16, 0.000000000000000000 ) ) ;
#8417=CARTESIAN_POINT ( 'NONE',  ( -1037.392967692957200, 114.2240391150264855, -113.1262384684098805 ) ) ;
#8425=CARTESIAN_POINT ( 'NONE',  ( -993.0619804577135028, 103.7129695969640579, -149.7857175106631757 ) ) ;
#8428=CARTESIAN_POINT ( 'NONE',  ( -1023.463303304735746, 92.47874188371233117, -154.2940595301281519 ) ) ;
#8434=CARTESIAN_POINT ( 'NONE',  ( -952.9945178120615310, 87.05516224832936700, -154.8742214401229660 ) ) ;
#8436=VERTEX_POINT ( 'NONE', #3410 ) ;
#8448=APPLICATION_CONTEXT ( 'automotive_design' ) ;
#8454=CARTESIAN_POINT ( 'NONE',  ( -1065.000000000007049, 56.89504896194527106, -107.9061927053324581 ) ) ;
#8455=CARTESIAN_POINT ( 'NONE',  ( -826.3398728605918677, 83.01019204304884624, -104.7054730589236016 ) ) ;
#8456=CARTESIAN_POINT ( 'NONE',  ( -976.2517683711890868, 35.25052392388818134, -126.6442663926290777 ) ) ;
#8457=CARTESIAN_POINT ( 'NONE',  ( -951.5459139781262365, 122.3346817490816676, -136.2353035311979852 ) ) ;
#8462=CARTESIAN_POINT ( 'NONE',  ( -1013.637332661006667, 62.09754518945625534, -103.3307627799637913 ) ) ;
#8468=CARTESIAN_POINT ( 'NONE',  ( -1018.154501869011938, 114.3413228342526082, -107.9061927053323870 ) ) ;
#8475=CARTESIAN_POINT ( 'NONE',  ( -1065.000000000000455, 107.1049510380560719, -107.9061927053323302 ) ) ;
#8484=CARTESIAN_POINT ( 'NONE',  ( -974.9912860506709649, 88.33816101283774458, -154.2940595301278108 ) ) ;
#8487=CARTESIAN_POINT ( 'NONE',  ( -1019.017691546887363, 99.44610047464912839, -152.5758913445291967 ) ) ;
#8491=CARTESIAN_POINT ( 'NONE',  ( -1023.860074334738101, 85.97273905232952984, -154.8742214401228523 ) ) ;
#8506=CARTESIAN_POINT ( 'NONE',  ( -1016.402231264574652, 68.39482517277133411, -99.57582448894554261 ) ) ;
#8507=CARTESIAN_POINT ( 'NONE',  ( -823.1752771847307031, 83.64233931405222222, -104.7482132693511403 ) ) ;
#8515=CARTESIAN_POINT ( 'NONE',  ( -1032.503061859599256, 50.81309391744463255, -107.9061927053326428 ) ) ;
#8518=CARTESIAN_POINT ( 'NONE',  ( -1011.051362836439694, 118.1813008219151868, -113.1262384684097952 ) ) ;
#8526=CARTESIAN_POINT ( 'NONE',  ( -1018.401127491270358, 110.2021201405460431, -103.3307627799636208 ) ) ;
#8530=CARTESIAN_POINT ( 'NONE',  ( -1024.691966601154036, 118.8493250655916142, -122.7172756069790580 ) ) ;
#8535=CARTESIAN_POINT ( 'NONE',  ( -974.3195816561885749, 116.7169707472886842, -141.4553492942758055 ) ) ;
#8547=CARTESIAN_POINT ( 'NONE',  ( -824.1700714248523809, 73.67466183167414329, -106.4959216872583028 ) ) ;
#8549=CARTESIAN_POINT ( 'NONE',  ( -1038.401083800579045, 57.54275223462362021, -149.7857175106632326 ) ) ;
#8558=CARTESIAN_POINT ( 'NONE',  ( -975.5821371384171243, 62.83201726680821508, -96.78565065507949328 ) ) ;
#8561=CARTESIAN_POINT ( 'NONE',  ( -854.0902776497799778, 23.28889115110665742, -122.7172756069793138 ) ) ;
#8569=CARTESIAN_POINT ( 'NONE',  ( -1057.693846703447207, 44.87596864925360052, -113.1262384684097100 ) ) ;
#8574=CARTESIAN_POINT ( 'NONE',  ( -852.8684863605125202, 118.0406360202081970, -113.1262384684093405 ) ) ;
#8579=VERTEX_POINT ( 'NONE', #5977 ) ;
#8583=CARTESIAN_POINT ( 'NONE',  ( -1021.777026427250121, 118.8177985574659346, -130.5712005305405228 ) ) ;
#8587=CARTESIAN_POINT ( 'NONE',  ( -1060.773655115450993, 112.4236047030758527, -118.7903414690679682 ) ) ;
#8591=CARTESIAN_POINT ( 'NONE',  ( -952.1456544189259148, 108.1568929870910836, -149.7857175106632042 ) ) ;
#8600=CARTESIAN_POINT ( 'NONE',  ( -974.4564103291385209, 111.0951925441807759, -146.0307792196441312 ) ) ;
#8609=CARTESIAN_POINT ( 'NONE',  ( -997.0443963278715955, 49.75991663364307271, -146.0307792196450691 ) ) ;
#8617=CARTESIAN_POINT ( 'NONE',  ( -976.1667687410277949, 38.51511931708004965, -136.2353035311986957 ) ) ;
#8618=ORIENTED_EDGE ( 'NONE', *, *, #941, .F. ) ;
#8620=CARTESIAN_POINT ( 'NONE',  ( -1032.260242496269029, 61.00429285198274698, -99.57582448894517313 ) ) ;
#8623=CARTESIAN_POINT ( 'NONE',  ( -976.2351830774960035, 35.86345807843989775, -130.5712005305402101 ) ) ;
#8626=CARTESIAN_POINT ( 'NONE',  ( -819.3316697785987799, 80.88429704961258437, -144.6519063719970006 ) ) ;
#8628=CARTESIAN_POINT ( 'NONE',  ( -828.3150505402204544, 76.46109783575887775, -154.6692737003968148 ) ) ;
#8631=CARTESIAN_POINT ( 'NONE',  ( -997.7839878466058963, 40.27522178589197921, -113.1262384684093547 ) ) ;
#8637=CARTESIAN_POINT ( 'NONE',  ( -951.7027691703317487, 118.7449601027236241, -107.9061927053324581 ) ) ;
#8647=CARTESIAN_POINT ( 'NONE',  ( -823.1749794181283733, 110.1592441374100844, -107.9061927053325292 ) ) ;
#8652=CARTESIAN_POINT ( 'NONE',  ( -1013.875822516560447, 120.2710389253235519, -122.7172756069789017 ) ) ;
#8654=CARTESIAN_POINT ( 'NONE',  ( -823.7697810748812799, 117.7733807739867871, -124.6807709998041531 ) ) ;
#8658=CARTESIAN_POINT ( 'NONE',  ( -1022.124201078499027, 113.7707856953084189, -141.4553492942762887 ) ) ;
#8673=CARTESIAN_POINT ( 'NONE',  ( -820.0492617104193869, 75.38478674231537013, -105.8049000242702533 ) ) ;
#8675=CARTESIAN_POINT ( 'NONE',  ( -853.9759289228051102, 31.63339360934212152, -141.4553492942759192 ) ) ;
#8686=CARTESIAN_POINT ( 'NONE',  ( -1028.259718048105469, 56.21337363619640115, -107.9061927053325434 ) ) ;
#8688=CARTESIAN_POINT ( 'NONE',  ( -819.4838385048408327, 81.17047855582200100, -104.6961160549178089 ) ) ;
#8689=CARTESIAN_POINT ( 'NONE',  ( -1048.334963668468163, 42.40858384259928471, -136.2353035311987242 ) ) ;
#8692=CARTESIAN_POINT ( 'NONE',  ( -824.1535707999410079, 73.67424315034676852, -154.6483812918586125 ) ) ;
#8693=ORIENTED_EDGE ( 'NONE', *, *, #4070, .T. ) ;
#8696=CARTESIAN_POINT ( 'NONE',  ( -1062.996098538733122, 47.98024286075321498, -118.7903414690683377 ) ) ;
#8704=CARTESIAN_POINT ( 'NONE',  ( -903.4746773471185861, 104.0883302344921475, -96.78565065507889642 ) ) ;
#8705=CARTESIAN_POINT ( 'NONE',  ( -795.0000000000038654, 109.8950841424301359, -136.2353035311980136 ) ) ;
#8708=CARTESIAN_POINT ( 'NONE',  ( -951.4198147059589701, 125.0824040815807194, -124.6807709998040252 ) ) ;
#8713=CARTESIAN_POINT ( 'NONE',  ( -1046.261572611719657, 104.4651992465226868, -146.0307792196445575 ) ) ;
#8716=( NAMED_UNIT ( * ) SI_UNIT ( $, .STERADIAN. ) SOLID_ANGLE_UNIT ( ) );
#8719=CARTESIAN_POINT ( 'NONE',  ( -1022.124201078499027, 113.7707856953084189, -141.4553492942762887 ) ) ;
#8727=CARTESIAN_POINT ( 'NONE',  ( -1047.844889418685170, 56.55730854968103927, -149.7857175106634315 ) ) ;
#8733=( LENGTH_UNIT ( ) NAMED_UNIT ( * ) SI_UNIT ( .MILLI., .METRE. ) );
#8740=CARTESIAN_POINT ( 'NONE',  ( -1014.107508992752514, 52.59077491224128664, -118.7903414690682951 ) ) ;
#8743=ORIENTED_EDGE ( 'NONE', *, *, #7308, .T. ) ;
#8752=CARTESIAN_POINT ( 'NONE',  ( -854.0803342822198374, 23.97549884981706825, -118.7903414690682808 ) ) ;
#8755=EDGE_CURVE ( 'NONE', #8579, #915, #7774, .T. ) ;
#8756=CARTESIAN_POINT ( 'NONE',  ( -853.1108559448483675, 99.60875591605646662, -99.57582448894477523 ) ) ;
#8763=CARTESIAN_POINT ( 'NONE',  ( -952.6992609796628813, 94.45070821374962122, -95.06748246947989855 ) ) ;
#8765=CARTESIAN_POINT ( 'NONE',  ( -991.8293279264742068, 119.7328159579556086, -136.2353035311976726 ) ) ;
#8769=CARTESIAN_POINT ( 'NONE',  ( -795.0000000000047748, 112.0000000000007532, -124.6807709998042384 ) ) ;
#8772=CARTESIAN_POINT ( 'NONE',  ( -1011.418100375194967, 110.6663390795549162, -146.0307792196444723 ) ) ;
#8784=CARTESIAN_POINT ( 'NONE',  ( -822.1919554870401043, 73.93830887977168231, -106.3769876045757599 ) ) ;
#8785=CARTESIAN_POINT ( 'NONE',  ( -953.5758047008371250, 72.53746257253824581, -152.5758913445294525 ) ) ;
#8786=CARTESIAN_POINT ( 'NONE',  ( -818.8285638327238303, 78.34153296655600229, -144.3462106687113646 ) ) ;
#8794=CARTESIAN_POINT ( 'NONE',  ( -928.4218612484578443, 59.99049470396625594, -130.5712005305400965 ) ) ;
#8798=CARTESIAN_POINT ( 'NONE',  ( -1063.013736978595944, 47.55218547899807646, -122.7172756069792570 ) ) ;
#8804=CARTESIAN_POINT ( 'NONE',  ( -827.8047116257844209, 75.62532219084948792, -154.6806748490619725 ) ) ;
#8808=CARTESIAN_POINT ( 'NONE',  ( -976.1667687410197232, 38.51511931707989334, -113.1262384684093263 ) ) ;
#8813=CARTESIAN_POINT ( 'NONE',  ( -903.8503739047830550, 115.2915043052427535, -103.3307627799633082 ) ) ;
#8819=CARTESIAN_POINT ( 'NONE',  ( -1061.468168685228193, 92.73456844357777129, -96.78565065507918064 ) ) ;
#8842=CARTESIAN_POINT ( 'NONE',  ( -821.2975544693643997, 74.34970510072432148, -106.2007125858228704 ) ) ;
#8843=CARTESIAN_POINT ( 'NONE',  ( -1065.000000000002956, 76.10956187831469322, -154.2940595301282087 ) ) ;
#8847=CARTESIAN_POINT ( 'NONE',  ( -828.8285638327251945, 78.34868723465601192, -94.76039716391075274 ) ) ;
#8855=CARTESIAN_POINT ( 'NONE',  ( -854.0803342822198374, 23.97549884981706825, -118.7903414690682808 ) ) ;
#8863=CARTESIAN_POINT ( 'NONE',  ( -795.0000000000020464, 54.10491585757070965, -113.1262384684093121 ) ) ;
#8868=CARTESIAN_POINT ( 'NONE',  ( -1031.476138302181198, 95.34216976508436403, -96.78565065507929432 ) ) ;
#8873=CARTESIAN_POINT ( 'NONE',  ( -1037.656130532294128, 99.96792753513312846, -99.57582448894522997 ) ) ;
#8875=CARTESIAN_POINT ( 'NONE',  ( -991.6207251904210125, 122.2801902404846714, -130.5712005305406080 ) ) ;
#8876=CARTESIAN_POINT ( 'NONE',  ( -974.1288507787422759, 124.2142274477005657, -124.6807709998040110 ) ) ;
#8881=EDGE_CURVE ( 'NONE', #140, #5809, #5117, .T. ) ;
#8890=EDGE_LOOP ( 'NONE', ( #252, #624 ) ) ;
#8896=CARTESIAN_POINT ( 'NONE',  ( -825.4444756108113097, 73.93131618268111538, -94.70140411087349719 ) ) ;
#8898=CARTESIAN_POINT ( 'NONE',  ( -997.0443963278715955, 49.75991663364307271, -146.0307792196450691 ) ) ;
#8903=CARTESIAN_POINT ( 'NONE',  ( -928.3598895237944362, 61.90886769853011629, -113.1262384684093831 ) ) ;
#8905=CARTESIAN_POINT ( 'NONE',  ( -826.3335398377358842, 83.00469051230240325, -95.17874826138289279 ) ) ;
#8915=CARTESIAN_POINT ( 'NONE',  ( -952.4132309232843454, 101.5728619241205450, -96.78565065507918064 ) ) ;
#8924=CARTESIAN_POINT ( 'NONE',  ( -1023.463303304735291, 92.47874188371200432, -95.06748246948023962 ) ) ;
#8927=CARTESIAN_POINT ( 'NONE',  ( -795.0000000000047748, 112.0000000000007532, -124.6807709998042384 ) ) ;
#8928=FACE_OUTER_BOUND ( 'NONE', #11751, .T. ) ;
#8931=CARTESIAN_POINT ( 'NONE',  ( -954.0688428831313104, 124.4732772249355577, -118.7903414690677693 ) ) ;
#8933=VECTOR ( 'NONE', #9682, 1000.000000000000000 ) ;
#8940=CARTESIAN_POINT ( 'NONE',  ( -991.5701548301636876, 122.8678427087060214, -124.6807709998040536 ) ) ;
#8947=B_SPLINE_CURVE_WITH_KNOTS ( 'NONE', 3,
 ( #11925, #10695, #9891, #2523, #12122, #3633, #9333, #7418, #7296, #11059, #2718, #873, #12186, #9396, #5793, #11306, #6611, #10618, #8654, #8769 ),
 .UNSPECIFIED., .F., .F.,
 ( 4, 1, 1, 1, 2, 1, 1, 1, 2, 2, 2, 2, 4 ),
 ( 0.000000000000000000, 0.04762575996673557022, 0.07143863995010346635, 0.09525151993347125146, 0.1428772799002068217, 0.1647615404280894369, 0.1757036706920307445, 0.1866458009559719411, 0.2085300614838545563, 0.4016963878702066726, 0.4307237013227157574, 0.6771470142487683308, 1.000000000000000000 ),
 .UNSPECIFIED. ) ;
#8954=CARTESIAN_POINT ( 'NONE',  ( -818.8614429351464423, 78.01598473359253205, -144.2826642275891800 ) ) ;
#8964=CARTESIAN_POINT ( 'NONE',  ( -1057.036663358150690, 58.23757105449725913, -149.7857175106634884 ) ) ;
#8974=CARTESIAN_POINT ( 'NONE',  ( -826.8798817544267195, 82.64869829037840532, -95.13516794514535491 ) ) ;
#8981=CARTESIAN_POINT ( 'NONE',  ( -1018.692594135739682, 105.1726068785156656, -99.57582448894508786 ) ) ;
#8988=SHAPE_REPRESENTATION_RELATIONSHIP ( 'NONE' , 'NONE' ,  #6213, #7064 ) ;
#8992=CARTESIAN_POINT ( 'NONE',  ( -1062.301584968951602, 67.66927912025059300, -96.78565065507969223 ) ) ;
#8995=CARTESIAN_POINT ( 'NONE',  ( -1021.743962174751232, 119.2557508373790824, -126.6442663926290209 ) ) ;
#9002=CARTESIAN_POINT ( 'NONE',  ( -821.6101090906096260, 83.16704697188406215, -95.16702136683898061 ) ) ;
#9005=CARTESIAN_POINT ( 'NONE',  ( -1010.922847972426780, 120.6260792194948550, -122.7172756069790296 ) ) ;
#9014=CARTESIAN_POINT ( 'NONE',  ( -853.5732225365131853, 62.99598188221416706, -154.2940595301278108 ) ) ;
#9024=CARTESIAN_POINT ( 'NONE',  ( -956.4793285278399253, 64.87563161486532692, -149.7857175106635452 ) ) ;
#9030=CARTESIAN_POINT ( 'NONE',  ( -828.5735930359926442, 80.28424781510358343, -94.89227360444822068 ) ) ;
#9043=CARTESIAN_POINT ( 'NONE',  ( -1015.209561144954137, 93.46821065761379543, -95.06748246948018277 ) ) ;
#9048=CARTESIAN_POINT ( 'NONE',  ( 0.000000000000000000, 0.000000000000000000, 0.000000000000000000 ) ) ;
#9054=CARTESIAN_POINT ( 'NONE',  ( -826.8818560538642259, 82.64726084648152948, -154.2265479354714444 ) ) ;
#9055=CARTESIAN_POINT ( 'NONE',  ( -927.8303129675875880, 79.95948428978934430, -96.78565065507952170 ) ) ;
#9064=CARTESIAN_POINT ( 'NONE',  ( -1028.611899521406940, 50.57492120214474340, -124.6807709998042384 ) ) ;
#9068=CARTESIAN_POINT ( 'NONE',  ( -823.7697810748812799, 117.7733807739867871, -124.6807709998041531 ) ) ;
#9078=CARTESIAN_POINT ( 'NONE',  ( -1065.000000000008868, 82.00000000000028422, -154.8742214401231081 ) ) ;
#9079=CARTESIAN_POINT ( 'NONE',  ( -824.6569351206132978, 73.74060470499460962, -142.8957018107301451 ) ) ;
#9082=CARTESIAN_POINT ( 'NONE',  ( -828.3247893467976155, 76.46300037722042475, -94.69171133721131639 ) ) ;
#9086=CARTESIAN_POINT ( 'NONE',  ( -854.0393178910245524, 26.93106345811121827, -136.2353035311989515 ) ) ;
#9092=VERTEX_POINT ( 'NONE', #10629 ) ;
#9103=B_SPLINE_CURVE_WITH_KNOTS ( 'NONE', 3,
 ( #949, #4, #5579, #831, #4604, #11324, #11213, #8376, #12143, #3656, #5639, #896, #7497, #3779, #7555, #2868, #6629, #10392, #8547, #1311, #2232, #2923, #8784, #6685, #8842, #4948, #7677, #8673, #2051, #6930, #10518, #2979, #10461, #5812, #10577, #7619 ),
 .UNSPECIFIED., .F., .F.,
 ( 4, 2, 2, 2, 2, 2, 2, 2, 2, 2, 2, 2, 2, 2, 2, 2, 2, 4 ),
 ( 0.01566607101767062554, 0.01666400919013300008, 0.01766194736259537462, 0.01865988553505774916, 0.01965782370752012370, 0.02065576187998249824, 0.02165370005244487278, 0.02215266913867606352, 0.02265163822490725426, 0.02364957639736996534, 0.02464751456983267641, 0.02564545274229539096, 0.02664339091475809856, 0.02764132908722081311, 0.02863926725968352072, 0.02963720543214623526, 0.03063514360460894634, 0.03163308177707165741 ),
 .UNSPECIFIED. ) ;
#9104=CARTESIAN_POINT ( 'NONE',  ( -1027.019426772557381, 78.04595964998433999, -95.06748246948046699 ) ) ;
#9116=CARTESIAN_POINT ( 'NONE',  ( -1038.283672687642365, 64.16172732404288581, -96.78565065507946485 ) ) ;
#9129=CARTESIAN_POINT ( 'NONE',  ( -974.1454360724308117, 123.6012932931490127, -118.7903414690677835 ) ) ;
#9131=CARTESIAN_POINT ( 'NONE',  ( -926.6866529579010603, 120.3119365386823034, -141.4553492942759760 ) ) ;
#9140=CARTESIAN_POINT ( 'NONE',  ( -955.6263874535649165, 86.32439835342530898, -154.8742214401227670 ) ) ;
#9141=CARTESIAN_POINT ( 'NONE',  ( -827.6116022231262832, 75.38889084172119226, -143.5581011396510007 ) ) ;
#9144=CARTESIAN_POINT ( 'NONE',  ( -1037.773541645230580, 93.34895244571352180, -152.5758913445289693 ) ) ;
#9148=CIRCLE ( 'NONE', #6590, 20.00000000000017053 ) ;
#9149=ORIENTED_EDGE ( 'NONE', *, *, #8755, .F. ) ;
#9150=CARTESIAN_POINT ( 'NONE',  ( -928.1401715909056520, 69.16346707077036626, -146.0307792196452965 ) ) ;
#9165=CARTESIAN_POINT ( 'NONE',  ( -1048.417899310732537, 40.17786091688628147, -130.5712005305406365 ) ) ;
#9172=CARTESIAN_POINT ( 'NONE',  ( -1038.158164256576356, 71.32123499372119113, -95.06748246948035330 ) ) ;
#9196=CARTESIAN_POINT ( 'NONE',  ( -1065.000000000003411, 111.6133447792289104, -118.7903414690678972 ) ) ;
#9203=ORIENTED_EDGE ( 'NONE', *, *, #7970, .F. ) ;
#9207=CARTESIAN_POINT ( 'NONE',  ( -1055.782959745576591, 85.17781532426890578, -154.2940595301287203 ) ) ;
#9208=CARTESIAN_POINT ( 'NONE',  ( -825.1469620822837214, 73.83976809224738247, -142.9404499552406094 ) ) ;
#9210=FACE_OUTER_BOUND ( 'NONE', #4407, .T. ) ;
#9211=CARTESIAN_POINT ( 'NONE',  ( -853.3345817150077437, 81.97571759610561060, -154.2940595301280098 ) ) ;
#9217=CARTESIAN_POINT ( 'NONE',  ( -902.6139906877482417, 77.75433758651681160, -152.5758913445294809 ) ) ;
#9234=CARTESIAN_POINT ( 'NONE',  ( -853.3345817150102448, 81.97571759610518427, -95.06748246948041015 ) ) ;
#9246=CARTESIAN_POINT ( 'NONE',  ( -1027.708477481198088, 65.70736702952430619, -99.57582448894528682 ) ) ;
#9261=CARTESIAN_POINT ( 'NONE',  ( -1037.348432443215870, 116.4729352038311987, -118.7903414690680961 ) ) ;
#9274=CARTESIAN_POINT ( 'NONE',  ( -1031.329434936838197, 101.6864263019769083, -149.7857175106636305 ) ) ;
#9276=ADVANCED_FACE ( 'NONE', ( #5055 ), #360, .T. ) ;
#9285=CARTESIAN_POINT ( 'NONE',  ( -927.6556653798983234, 86.18751778479050074, -154.2940595301282656 ) ) ;
#9300=CARTESIAN_POINT ( 'NONE',  ( -1019.723937646958007, 86.79129919622097589, -94.48732055948626396 ) ) ;
#9303=CARTESIAN_POINT ( 'NONE',  ( -1063.013736978594579, 47.55218547899811199, -126.6442663926291914 ) ) ;
#9304=CARTESIAN_POINT ( 'NONE',  ( -820.4056028115179515, 82.32260517263534894, -144.6785023965176435 ) ) ;
#9311=CARTESIAN_POINT ( 'NONE',  ( -1057.299536696272526, 52.76571712355550403, -103.3307627799637487 ) ) ;
#9329=ADVANCED_FACE ( 'NONE', ( #602 ), #5414, .F. ) ;
#9333=CARTESIAN_POINT ( 'NONE',  ( -1024.691966601152672, 118.8493250655916142, -124.6807709998039400 ) ) ;
#9336=CARTESIAN_POINT ( 'NONE',  ( -1061.276350651670782, 98.40484402385492047, -149.7857175106635452 ) ) ;
#9339=CARTESIAN_POINT ( 'NONE',  ( -1031.476138302183244, 95.34216976508434982, -152.5758913445290830 ) ) ;
#9345=CARTESIAN_POINT ( 'NONE',  ( -1012.527716518106786, 86.38194213450564973, -154.8742214401233070 ) ) ;
#9349=ORIENTED_EDGE ( 'NONE', *, *, #2065, .F. ) ;
#9350=CARTESIAN_POINT ( 'NONE',  ( -828.7978644797699417, 79.31746325908761719, -144.5027040960659974 ) ) ;
#9352=CARTESIAN_POINT ( 'NONE',  ( -1038.595419435783924, 46.89684673038589580, -141.4553492942758623 ) ) ;
#9365=CARTESIAN_POINT ( 'NONE',  ( -956.7203770923135835, 58.97922774997691420, -103.3307627799636919 ) ) ;
#9368=CARTESIAN_POINT ( 'NONE',  ( -928.4368846968627622, 59.55532739646334051, -122.7172756069790154 ) ) ;
#9376=CARTESIAN_POINT ( 'NONE',  ( -1038.595419435790973, 46.89684673038605922, -107.9061927053327850 ) ) ;
#9389=CARTESIAN_POINT ( 'NONE',  ( -1031.000617048998265, 115.3267894020684992, -113.1262384684098521 ) ) ;
#9396=CARTESIAN_POINT ( 'NONE',  ( -954.0441199534440102, 124.9954171138387977, -124.6807709998039115 ) ) ;
#9399=CARTESIAN_POINT ( 'NONE',  ( -955.3297122972861644, 93.84065249268903131, -154.2940595301280950 ) ) ;
#9402=CARTESIAN_POINT ( 'NONE',  ( -1023.078931369431530, 98.73915068298377662, -152.5758913445292535 ) ) ;
#9407=CARTESIAN_POINT ( 'NONE',  ( -820.4595805503685142, 72.64106675864371709, -154.8742214401225397 ) ) ;
#9415=CARTESIAN_POINT ( 'NONE',  ( -1016.863910020547223, 59.13213530333427315, -141.4553492942757487 ) ) ;
#9426=CARTESIAN_POINT ( 'NONE',  ( -1062.493403002516516, 61.99900353997416147, -99.57582448894515892 ) ) ;
#9427=CARTESIAN_POINT ( 'NONE',  ( -825.4402961394322347, 83.41886444745711060, -104.7307635270716304 ) ) ;
#9429=CARTESIAN_POINT ( 'NONE',  ( -1048.417899310732537, 40.17786091688628147, -130.5712005305406365 ) ) ;
#9436=CARTESIAN_POINT ( 'NONE',  ( -927.9936929689729368, 74.21188826700399943, -99.57582448894522997 ) ) ;
#9438=DIRECTION ( 'NONE',  ( 1.000000000000000000, 0.000000000000000000, 0.000000000000000000 ) ) ;
#9451=FACE_BOUND ( 'NONE', #6334, .T. ) ;
#9457=CARTESIAN_POINT ( 'NONE',  ( -822.2439855206093853, 97.57287547056431265, -149.7857175106634600 ) ) ;
#9468=CARTESIAN_POINT ( 'NONE',  ( -828.3910170805090729, 80.72627522873344219, -144.6407408995351318 ) ) ;
#9471=CARTESIAN_POINT ( 'NONE',  ( -997.4616017999776432, 44.34671234275830187, -141.4553492942759476 ) ) ;
#9483=CARTESIAN_POINT ( 'NONE',  ( -818.6751755801135459, 47.70925804672316417, -99.57582448894514471 ) ) ;
#9485=CARTESIAN_POINT ( 'NONE',  ( -1028.611899521407167, 50.57492120214475761, -126.6442663926292340 ) ) ;
#9493=CARTESIAN_POINT ( 'NONE',  ( -795.0000000000050022, 56.89504896194521422, -107.9061927053325860 ) ) ;
#9506=CARTESIAN_POINT ( 'NONE',  ( -992.1517139731023462, 115.6613254010895986, -107.9061927053323870 ) ) ;
#9508=CARTESIAN_POINT ( 'NONE',  ( -1021.913416468810851, 116.8879375517085464, -136.2353035311978431 ) ) ;
#9511=CARTESIAN_POINT ( 'NONE',  ( -904.2101318205999405, 125.2895275102983419, -124.6807709998041531 ) ) ;
#9513=DIRECTION ( 'NONE',  ( 0.000000000000000000, 1.000000000000000000, 6.938893903907169213E-16 ) ) ;
#9515=DIRECTION ( 'NONE',  ( 0.000000000000000000, 5.522905491341382306E-16, 1.000000000000000000 ) ) ;
#9516=CARTESIAN_POINT ( 'NONE',  ( -992.5689194452182846, 110.2481211102048491, -146.0307792196443870 ) ) ;
#9522=CARTESIAN_POINT ( 'NONE',  ( -954.7734463792789938, 107.7731650919854758, -149.7857175106632042 ) ) ;
#9530=CARTESIAN_POINT ( 'NONE',  ( -1057.299536696276846, 52.76571712355565325, -146.0307792196449554 ) ) ;
#9535=FILL_AREA_STYLE ('',( #5759 ) ) ;
#9536=CARTESIAN_POINT ( 'NONE',  ( -957.1839320239870403, 48.17551948191491817, -130.5712005305400112 ) ) ;
#9542=CARTESIAN_POINT ( 'NONE',  ( -953.5758047008322364, 72.53746257253780527, -96.78565065507940801 ) ) ;
#9543=CARTESIAN_POINT ( 'NONE',  ( -827.8090925714953983, 81.71768170412181576, -104.6809152895179693 ) ) ;
#9544=CARTESIAN_POINT ( 'NONE',  ( -997.9925905826634107, 37.72784750336339954, -130.5712005305403238 ) ) ;
#9546=CARTESIAN_POINT ( 'NONE',  ( -974.2138504089066373, 120.9496320545085695, -136.2353035311977010 ) ) ;
#9551=CARTESIAN_POINT ( 'NONE',  ( -1038.664246639915291, 43.28664065472965206, -113.1262384684093405 ) ) ;
#9557=CARTESIAN_POINT ( 'NONE',  ( -992.1517139731023462, 115.6613254010895986, -107.9061927053323870 ) ) ;
#9568=CARTESIAN_POINT ( 'NONE',  ( -852.8684863605125202, 118.0406360202081970, -113.1262384684093405 ) ) ;
#9569=CARTESIAN_POINT ( 'NONE',  ( -1037.348432443219735, 116.4729352038311987, -130.5712005305406080 ) ) ;
#9572=CARTESIAN_POINT ( 'NONE',  ( -795.0000000000046612, 112.0000000000007532, -122.7172756069791717 ) ) ;
#9579=CARTESIAN_POINT ( 'NONE',  ( -904.0006525278439540, 119.6095687608908378, -141.4553492942759760 ) ) ;
#9586=CARTESIAN_POINT ( 'NONE',  ( -992.1517139731079169, 115.6613254010897123, -141.4553492942762318 ) ) ;
#9592=CARTESIAN_POINT ( 'NONE',  ( -1028.007066121607295, 60.50166182213178701, -146.0307792196450123 ) ) ;
#9597=SURFACE_SIDE_STYLE ('',( #10763 ) ) ;
#9601=ORIENTED_EDGE ( 'NONE', *, *, #2463, .F. ) ;
#9605=CARTESIAN_POINT ( 'NONE',  ( -1038.506348936316726, 51.71309463382168303, -103.3307627799636350 ) ) ;
#9606=CARTESIAN_POINT ( 'NONE',  ( -825.1278902672622735, 83.51360356663572304, -104.7380248171176618 ) ) ;
#9609=CARTESIAN_POINT ( 'NONE',  ( -826.3315746005818028, 74.34282231245687456, -154.6710292045187032 ) ) ;
#9611=EDGE_CURVE ( 'NONE', #9730, #140, #3977, .T. ) ;
#9613=CARTESIAN_POINT ( 'NONE',  ( -1032.644706488208840, 45.21923725197571997, -118.7903414690683519 ) ) ;
#9623=CARTESIAN_POINT ( 'NONE',  ( -1014.632462699974781, 105.5176738732103132, -99.57582448894522997 ) ) ;
#9625=CARTESIAN_POINT ( 'NONE',  ( -974.1454360724337675, 123.6012932931491690, -130.5712005305403238 ) ) ;
#9628=CARTESIAN_POINT ( 'NONE',  ( -852.8175266017511831, 121.6828083272127685, -124.6807709998041247 ) ) ;
#9634=CARTESIAN_POINT ( 'NONE',  ( -795.0000000000046612, 103.3499740386315864, -146.0307792196441312 ) ) ;
#9643=CARTESIAN_POINT ( 'NONE',  ( -1011.418100375194967, 110.6663390795549162, -146.0307792196444723 ) ) ;
#9655=CARTESIAN_POINT ( 'NONE',  ( -1065.000000000007731, 60.65002596136951496, -146.0307792196448986 ) ) ;
#9660=SURFACE_STYLE_USAGE ( .BOTH. , #9597 ) ;
#9666=CARTESIAN_POINT ( 'NONE',  ( -1025.943122242217214, 53.12767954719360830, -118.7903414690682524 ) ) ;
#9669=CARTESIAN_POINT ( 'NONE',  ( -1021.483947769362658, 56.15424078096121008, -136.2353035311990368 ) ) ;
#9672=CARTESIAN_POINT ( 'NONE',  ( -825.1261283413638239, 73.83457159616112619, -154.6564883458196107 ) ) ;
#9676=CARTESIAN_POINT ( 'NONE',  ( -1048.417899310738221, 40.17786091688638095, -118.7903414690680250 ) ) ;
#9679=CARTESIAN_POINT ( 'NONE',  ( -1037.656130532294128, 99.96792753513312846, -99.57582448894522997 ) ) ;
#9682=DIRECTION ( 'NONE',  ( 0.000000000000000000, 5.522905491341382306E-16, 1.000000000000000000 ) ) ;
#9684=CARTESIAN_POINT ( 'NONE',  ( -1046.676250823070177, 92.10743237175765330, -96.78565065507946485 ) ) ;
#9689=CARTESIAN_POINT ( 'NONE',  ( -954.0441199534440102, 124.9954171138387977, -124.6807709998039115 ) ) ;
#9694=CARTESIAN_POINT ( 'NONE',  ( -818.8285638327242850, 78.67432280806571043, -264.6807709998050200 ) ) ;
#9695=CARTESIAN_POINT ( 'NONE',  ( -1014.007272717915953, 117.9006809476442896, -136.2353035311982126 ) ) ;
#9705=CARTESIAN_POINT ( 'NONE',  ( -1061.104375862961888, 103.3839434440459968, -146.0307792196447565 ) ) ;
#9713=CARTESIAN_POINT ( 'NONE',  ( -1013.392840968502924, 67.31954129910421614, -149.7857175106636873 ) ) ;
#9722=CARTESIAN_POINT ( 'NONE',  ( -976.2351830775012331, 35.86345807843999012, -118.7903414690679824 ) ) ;
#9726=CARTESIAN_POINT ( 'NONE',  ( -825.8938804283657191, 83.23078805786300904, -95.20686423277604149 ) ) ;
#9728=CARTESIAN_POINT ( 'NONE',  ( -820.5243268950206357, 74.90756738765448119, -154.6705515957940520 ) ) ;
#9730=VERTEX_POINT ( 'NONE', #7012 ) ;
#9733=CARTESIAN_POINT ( 'NONE',  ( -854.0902776497799778, 23.28889115110665742, -122.7172756069793138 ) ) ;
#9736=CARTESIAN_POINT ( 'NONE',  ( -795.0000000000002274, 98.77454568802498613, -99.57582448894500260 ) ) ;
#9742=CARTESIAN_POINT ( 'NONE',  ( -821.6815100408621220, 89.78153722040228502, -96.78565065507908116 ) ) ;
#9744=CARTESIAN_POINT ( 'NONE',  ( -852.8684863605087685, 118.0406360202081970, -136.2353035311977862 ) ) ;
#9755=ORIENTED_EDGE ( 'NONE', *, *, #4070, .F. ) ;
#9770=CARTESIAN_POINT ( 'NONE',  ( -1016.123300349502756, 74.17810748283176281, -152.5758913445294525 ) ) ;
#9781=CARTESIAN_POINT ( 'NONE',  ( -1028.611899521406713, 50.57492120214472919, -122.7172756069792428 ) ) ;
#9784=CARTESIAN_POINT ( 'NONE',  ( -828.3149917726251488, 80.88765617246495765, -94.94636425413492020 ) ) ;
#9791=CARTESIAN_POINT ( 'NONE',  ( -1038.719578313837474, 40.52245044769760085, -126.6442663926297740 ) ) ;
#9797=CARTESIAN_POINT ( 'NONE',  ( -795.0000000000070486, 103.3499740386316859, -103.3307627799634218 ) ) ;
#9804=CARTESIAN_POINT ( 'NONE',  ( -821.0802431487063586, 81.36881375820571805, -95.06748246948008330 ) ) ;
#9807=CARTESIAN_POINT ( 'NONE',  ( -1060.756016675586807, 112.8516620848305934, -124.6807709998040821 ) ) ;
#9810=CARTESIAN_POINT ( 'NONE',  ( -1030.944970944895431, 117.4714819019837222, -118.7903414690680535 ) ) ;
#9820=CARTESIAN_POINT ( 'NONE',  ( -1037.337636019038882, 116.9882293220588991, -124.6807709998043521 ) ) ;
#9827=CARTESIAN_POINT ( 'NONE',  ( -1047.392513188124212, 70.23666496464454667, -154.2940595301285214 ) ) ;
#9836=CARTESIAN_POINT ( 'NONE',  ( -1062.493403002509012, 61.99900353997395541, -149.7857175106634315 ) ) ;
#9844=CARTESIAN_POINT ( 'NONE',  ( -1048.438004920983758, 39.66697241395321782, -122.7172756069793138 ) ) ;
#9860=CARTESIAN_POINT ( 'NONE',  ( -952.1456544189251190, 108.1568929870907141, -99.57582448894486049 ) ) ;
#9871=CARTESIAN_POINT ( 'NONE',  ( -1037.773541645229670, 93.34895244571353601, -96.78565065507908116 ) ) ;
#9873=CARTESIAN_POINT ( 'NONE',  ( -1065.000000000006594, 112.0000000000007105, -124.6807709998041531 ) ) ;
#9879=CARTESIAN_POINT ( 'NONE',  ( -1065.000000000003865, 52.00000000000021316, -124.6807709998039826 ) ) ;
#9882=CARTESIAN_POINT ( 'NONE',  ( -820.5220565119172988, 82.43903826675141033, -95.06393426016371961 ) ) ;
#9885=CARTESIAN_POINT ( 'NONE',  ( -1013.875822516558969, 120.2710389253236940, -126.6442663926291061 ) ) ;
#9891=CARTESIAN_POINT ( 'NONE',  ( -1054.380968608931425, 114.0683136310379524, -124.6807709998043663 ) ) ;
#9895=CARTESIAN_POINT ( 'NONE',  ( -819.4917226271898016, 76.16439187810770761, -94.68015410868913762 ) ) ;
#9898=CARTESIAN_POINT ( 'NONE',  ( -954.2862664537763067, 55.36536439393486830, -141.4553492942758908 ) ) ;
#9903=CARTESIAN_POINT ( 'NONE',  ( -1065.000000000006594, 52.38665522077229042, -118.7903414690683945 ) ) ;
#9909=CARTESIAN_POINT ( 'NONE',  ( -1025.976186494711783, 52.68972726728017619, -126.6442663926293193 ) ) ;
#9915=CARTESIAN_POINT ( 'NONE',  ( -1046.909978542194949, 84.99913997988220160, -95.06748246948046699 ) ) ;
#9924=CARTESIAN_POINT ( 'NONE',  ( -795.0000000000004547, 76.10956187831470743, -95.06748246948018277 ) ) ;
#9936=CARTESIAN_POINT ( 'NONE',  ( -822.2117862628927014, 83.41691093530795342, -95.20655667354223795 ) ) ;
#9939=CARTESIAN_POINT ( 'NONE',  ( -1060.756016675586807, 112.8516620848305934, -124.6807709998040821 ) ) ;
#9950=CARTESIAN_POINT ( 'NONE',  ( -819.8389179520123662, 63.91331975908080665, -154.2940595301278677 ) ) ;
#9959=CARTESIAN_POINT ( 'NONE',  ( -822.0694275022420925, 73.99112643935335143, -94.71034476858436335 ) ) ;
#9961=CARTESIAN_POINT ( 'NONE',  ( -853.8938961404190877, 37.86297855175782701, -146.0307792196449554 ) ) ;
#9978=( GEOMETRIC_REPRESENTATION_CONTEXT ( 3 ) GLOBAL_UNCERTAINTY_ASSIGNED_CONTEXT ( ( #212 ) ) GLOBAL_UNIT_ASSIGNED_CONTEXT ( ( #7205, #11898, #8716 ) ) REPRESENTATION_CONTEXT ( 'NONE', 'WORKASPACE' ) );
#9979=CARTESIAN_POINT ( 'NONE',  ( -1056.430032577878137, 71.19035303699463668, -95.06748246948046699 ) ) ;
#9989=CARTESIAN_POINT ( 'NONE',  ( -1047.626240907246483, 63.12837257276869707, -96.78565065507969223 ) ) ;
#9994=CARTESIAN_POINT ( 'NONE',  ( -1024.722591077092829, 118.3980260646366958, -118.7903414690678403 ) ) ;
#10002=CARTESIAN_POINT ( 'NONE',  ( -1013.875822516560447, 120.2710389253235519, -122.7172756069789017 ) ) ;
#10014=CARTESIAN_POINT ( 'NONE',  ( -955.9230626098308221, 78.80814421416198456, -154.2940595301282372 ) ) ;
#10018=CARTESIAN_POINT ( 'NONE',  ( -826.8800118742810810, 74.69996070206661898, -94.68424396577464108 ) ) ;
#10022=CARTESIAN_POINT ( 'NONE',  ( -1062.810894920117335, 52.92335929224806534, -141.4553492942755781 ) ) ;
#10032=ORIENTED_EDGE ( 'NONE', *, *, #8881, .F. ) ;
#10037=CARTESIAN_POINT ( 'NONE',  ( -954.5692209181572707, 49.02792041507773746, -126.6442663926294045 ) ) ;
#10042=CARTESIAN_POINT ( 'NONE',  ( -1012.226803665789134, 93.06815595962675047, -95.06748246948018277 ) ) ;
#10049=CARTESIAN_POINT ( 'NONE',  ( -822.5362431349451526, 83.50721794775202511, -154.1394416282527970 ) ) ;
#10050=CARTESIAN_POINT ( 'NONE',  ( -1031.794838716553841, 81.34535957697958963, -94.48732055948609343 ) ) ;
#10052=CARTESIAN_POINT ( 'NONE',  ( -1065.000000000003865, 112.0000000000008527, -126.6442663926290493 ) ) ;
#10061=CARTESIAN_POINT ( 'NONE',  ( -951.4198147059590838, 125.0824040815807194, -122.7172756069790864 ) ) ;
#10062=CARTESIAN_POINT ( 'NONE',  ( -795.0000000000043201, 82.00000000000039790, -124.6807709998041105 ) ) ;
#10070=CARTESIAN_POINT ( 'NONE',  ( -955.0423082396526979, 101.0797422464698769, -152.5758913445288272 ) ) ;
#10074=CARTESIAN_POINT ( 'NONE',  ( -955.3297122972861644, 93.84065249268903131, -154.2940595301280950 ) ) ;
#10079=ORIENTED_EDGE ( 'NONE', *, *, #7525, .T. ) ;
#10081=CARTESIAN_POINT ( 'NONE',  ( -1028.007066121607295, 60.50166182213178701, -146.0307792196450123 ) ) ;
#10085=ORIENTED_EDGE ( 'NONE', *, *, #2424, .F. ) ;
#10094=CARTESIAN_POINT ( 'NONE',  ( -1062.996098538724254, 47.98024286075312261, -130.5712005305402101 ) ) ;
#10099=CARTESIAN_POINT ( 'NONE',  ( -955.6263874535618470, 86.32439835342511003, -94.48732055948597974 ) ) ;
#10108=CARTESIAN_POINT ( 'NONE',  ( -820.7809001343154023, 82.65155347377678652, -154.2690219959281421 ) ) ;
#10109=CARTESIAN_POINT ( 'NONE',  ( -995.4135022096149896, 71.70161378084165449, -95.06748246948046699 ) ) ;
#10122=CARTESIAN_POINT ( 'NONE',  ( -1045.864486809339951, 115.5688325305733741, -122.7172756069790438 ) ) ;
#10123=CARTESIAN_POINT ( 'NONE',  ( -1065.000000000003865, 52.00000000000021316, -124.6807709998039826 ) ) ;
#10132=CARTESIAN_POINT ( 'NONE',  ( -1055.176328965298808, 98.13059730676609149, -149.7857175106632326 ) ) ;
#10144=CARTESIAN_POINT ( 'NONE',  ( -1020.430183747032629, 74.13649791779326392, -152.5758913445297651 ) ) ;
#10157=CARTESIAN_POINT ( 'NONE',  ( -1028.581275045468146, 51.02622020309988216, -130.5712005305406080 ) ) ;
#10163=CARTESIAN_POINT ( 'NONE',  ( -819.8389179520128209, 63.91331975908082086, -95.06748246948014014 ) ) ;
#10166=CARTESIAN_POINT ( 'NONE',  ( -795.0000000000047748, 52.00000000000024158, -122.7172756069790154 ) ) ;
#10175=CARTESIAN_POINT ( 'NONE',  ( -1015.517346982276649, 86.95624952299064603, -94.48732055948629238 ) ) ;
#10189=CARTESIAN_POINT ( 'NONE',  ( -951.4198147059589701, 125.0824040815807194, -124.6807709998040252 ) ) ;
#10199=CARTESIAN_POINT ( 'NONE',  ( -903.4746773471192682, 104.0883302344920480, -152.5758913445288272 ) ) ;
#10203=CARTESIAN_POINT ( 'NONE',  ( -795.0000000000080718, 93.55451860843929524, -152.5758913445291398 ) ) ;
#10210=CARTESIAN_POINT ( 'NONE',  ( -1024.641217300042399, 73.20632742167555307, -152.5758913445296230 ) ) ;
#10229=CARTESIAN_POINT ( 'NONE',  ( -1023.463303304735291, 92.47874188371200432, -95.06748246948023962 ) ) ;
#10232=CARTESIAN_POINT ( 'NONE',  ( -928.4368846968637854, 59.55532739646334051, -126.6442663926292056 ) ) ;
#10240=CARTESIAN_POINT ( 'NONE',  ( -928.1401715908999677, 69.16346707076998257, -103.3307627799636919 ) ) ;
#10242=DIRECTION ( 'NONE',  ( 1.000000000000000000, 0.000000000000000000, 0.000000000000000000 ) ) ;
#10255=CARTESIAN_POINT ( 'NONE',  ( -1011.211222789223370, 114.9684118750912489, -107.9061927053323870 ) ) ;
#10266=CARTESIAN_POINT ( 'NONE',  ( -853.4539021257704690, 72.48584973916007357, -154.8742214401226818 ) ) ;
#10269=CYLINDRICAL_SURFACE ( 'NONE', #673, 20.00000000000017053 ) ;
#10274=CARTESIAN_POINT ( 'NONE',  ( -1019.723937646960849, 86.79129919622100431, -154.8742214401232502 ) ) ;
#10277=CARTESIAN_POINT ( 'NONE',  ( -1057.521967982373098, 48.25222617153974625, -141.4553492942758623 ) ) ;
#10282=VERTEX_POINT ( 'NONE', #1459 ) ;
#10284=B_SPLINE_SURFACE_WITH_KNOTS ( 'NONE', 3, 3, ( 
 ( #6851, #10616, #3823, #989, #2904, #5854, #11427, #4929, #7597, #1115, #3762, #2843, #4986, #9689, #8708, #4867, #9511, #9628, #7712, #2960 ),
 ( #11365, #7536, #11304, #6609, #1979, #6723, #8530, #4010, #6668, #8652, #2159, #5922, #1175, #10499, #1056, #5791, #7778, #1232, #3021, #9572 ),
 ( #4814, #8587, #10371, #109, #3137, #9810, #9994, #10738, #7027, #10917, #8025, #4075, #7907, #8931, #7844, #11618, #10674, #1293, #1465, #464 ),
 ( #8086, #7152, #4188, #3193, #1350, #5114, #11736, #2338, #6107, #2450, #8518, #6771, #6656, #10487, #214, #1163, #3936, #8574, #5724, #3872 ),
 ( #5844, #4856, #98, #5778, #1041, #7644, #5604, #3996, #8468, #11413, #3068, #9557, #1103, #11541, #8637, #1840, #3011, #4694, #6837, #12230 ),
 ( #5205, #4299, #1444, #10786, #8068, #272, #3123, #2262, #5097, #4063, #10606, #10664, #7828, #1337, #6033, #4121, #8813, #2144, #6895, #9797 ),
 ( #1217, #1278, #7895, #11603, #9679, #443, #5909, #3351, #8981, #3236, #2201, #5968, #512, #5036, #9860, #3179, #11840, #8756, #11662, #9736 ),
 ( #1391, #335, #6956, #10724, #4975, #8868, #393, #4172, #7949, #11721, #7015, #2323, #6092, #5153, #8915, #4236, #8010, #11780, #3296, #7071 ),
 ( #10842, #2376, #6147, #9915, #11028, #6328, #6455, #10229, #7197, #9043, #10042, #5458, #2558, #12087, #7326, #11091, #1509, #9234, #1765, #5270 ),
 ( #7133, #2493, #2430, #1572, #4548, #6211, #5526, #842, #9300, #2616, #4614, #581, #11891, #10099, #1632, #4358, #10899, #10966, #8128, #5393 ),
 ( #643, #5333, #9979, #3406, #9172, #6270, #9104, #4418, #8195, #11958, #3474, #776, #4485, #12156, #8258, #12017, #3533, #6392, #10163, #1698 ),
 ( #8324, #3598, #7387, #11158, #2684, #4790, #11280, #10528, #10406, #10473, #2993, #7689, #8558, #2008, #9542, #1947, #12212, #5652, #3920, #15 ),
 ( #6520, #9426, #5764, #11335, #962, #8620, #10287, #4676, #1890, #8506, #2876, #4734, #2070, #2752, #3792, #6641, #5708, #7566, #9483, #7444 ),
 ( #5827, #79, #1021, #3857, #9605, #7630, #1088, #6582, #11399, #2936, #11462, #5589, #6754, #9365, #1827, #6699, #910, #4842, #137, #1148 ),
 ( #8454, #3735, #7509, #2811, #10346, #4900, #8686, #3671, #11226, #2246, #7813, #11709, #10650, #11522, #10590, #3979, #1205, #7748, #2188, #10830 ),
 ( #5142, #3051, #3223, #11587, #7999, #5889, #317, #11647, #11768, #3283, #257, #2131, #3108, #10770, #4105, #8903, #4047, #1320, #194, #6821 ),
 ( #9903, #430, #5080, #5954, #6077, #4162, #7877, #9666, #6881, #4962, #8740, #5196, #9722, #6940, #1259, #4220, #5020, #8855, #2369, #7058 ),
 ( #10709, #8798, #6015, #9844, #6136, #7000, #9781, #7936, #3166, #382, #2307, #1437, #1379, #5592, #7632, #9368, #912, #8561, #5654, #10166 ),
 ( #1700, #9303, #3795, #5461, #1025, #82, #9485, #10349, #3859, #8327, #6458, #4678, #8456, #12089, #4552, #10232, #1768, #12214, #3738, #7512 ),
 ( #5528, #11282, #2814, #9429, #964, #4737, #7568, #11337, #2879, #10409, #1950, #9544, #8623, #11589, #7691, #6756, #139, #5829, #5957, #7751 ),
 ( #2072, #11524, #1150, #8689, #320, #6824, #10592, #5892, #9669, #6018, #259, #6883, #3168, #6943, #8377, #3657, #3725, #5698, #764, #8316 ),
 ( #2739, #6507, #10277, #11326, #9352, #11271, #6571, #1878, #5641, #9415, #950, #9471, #11573, #4030, #2980, #7802, #4949, #8675, #6871, #4832 ),
 ( #9655, #5754, #9530, #3158, #7679, #3101, #9592, #2233, #2924, #2053, #1074, #8609, #10640, #129, #6686, #3905, #3846, #7865, #5814, #10462 ),
 ( #6741, #1137, #4887, #8727, #8549, #11449, #67, #10519, #6931, #7620, #9713, #11387, #2179, #182, #309, #1996, #3965, #7734, #4095, #11639 ),
 ( #11508, #3037, #5941, #6807, #1251, #10579, #5875, #4778, #2117, #9770, #6000, #5006, #1197, #245, #8785, #10696, #485, #11694, #11757, #5065 ),
 ( #8843, #2358, #11812, #9827, #6246, #3328, #2407, #2527, #614, #3381, #7108, #3209, #10871, #10014, #5305, #4332, #6184, #9014, #9950, #1488 ),
 ( #9078, #6985, #8102, #10758, #4389, #8162, #2291, #6060, #1367, #5428, #5362, #743, #7482, #9140, #4707, #3768, #935, #10266, #3566, #3705 ),
 ( #1740, #679, #9207, #1601, #4454, #2847, #12054, #4585, #6360, #2785, #4521, #11199, #8484, #9399, #12190, #8359, #11992, #12125, #6550, #1859 ),
 ( #3636, #1797, #8299, #6429, #8232, #10317, #3507, #7357, #11309, #11127, #7421, #5238, #5561, #10070, #2652, #7299, #10199, #5621, #11063, #7541 ),
 ( #2588, #9336, #10132, #1666, #5501, #9274, #2721, #813, #6491, #877, #4649, #8425, #2038, #113, #8591, #10378, #11371, #5796, #9457, #995 ),
 ( #3891, #3827, #5680, #8713, #1918, #6614, #4992, #11494, #7602, #2911, #8772, #9516, #5859, #11432, #7849, #4760, #7662, #6673, #10443, #9634 ),
 ( #1119, #1182, #5927, #10621, #6789, #4935, #229, #8658, #1983, #2965, #6858, #6727, #8535, #50, #10503, #4016, #9579, #169, #11559, #5740 ),
 ( #3951, #7717, #10563, #2106, #293, #1060, #7783, #3085, #2166, #9695, #2012, #2757, #9546, #4681, #8457, #10308, #11115, #6601, #4440, #11094 ),
 ( #3132, #1001, #60, #6905, #7903, #11673, #3187, #6963, #4769, #2916, #10452, #8875, #11729, #3244, #1226, #6104, #1402, #7839, #456, #1809 ),
 ( #825, #1002, #5634, #940, #4876, #2852, #361, #4145, #410, #9885, #234, #4020, #7788, #1242, #6863, #2349, #8036, #1416, #3318, #7917 ),
 ( #1359, #300, #1186, #11566, #9820, #5127, #3093, #4199, #5179, #10630, #2171, #8940, #6977, #7100, #11682, #10748, #4941, #6119, #3148, #11802 ) ),
 .UNSPECIFIED., .T., .F., .F.,
 ( 4, 1, 1, 1, 1, 1, 1, 1, 1, 1, 1, 1, 1, 1, 1, 1, 2, 1, 1, 1, 1, 1, 1, 1, 1, 1, 1, 1, 1, 1, 1, 1, 4 ),
 ( 4, 1, 1, 1, 2, 1, 1, 1, 2, 2, 2, 2, 4 ),
 ( 0.000000000000000000, 0.03125000000000000000, 0.06250000000000000000, 0.09375000000000000000, 0.1250000000000000000, 0.1562500000000000000, 0.1875000000000000000, 0.2187500000000000000, 0.2500000000000000000, 0.2812500000000000000, 0.3125000000000000000, 0.3437500000000000000, 0.3750000000000000000, 0.4062500000000000000, 0.4375000000000000000, 0.4687500000000000000, 0.5000000000000000000, 0.5312500000000000000, 0.5625000000000000000, 0.5937500000000000000, 0.6250000000000000000, 0.6562500000000000000, 0.6875000000000000000, 0.7187500000000000000, 0.7500000000000000000, 0.7812500000000000000, 0.8125000000000000000, 0.8437500000000000000, 0.8750000000000000000, 0.9062500000000000000, 0.9375000000000000000, 0.9687500000000000000, 1.000000000000000000 ),
 ( 0.000000000000000000, 0.04762575996673557022, 0.07143863995010346635, 0.09525151993347125146, 0.1428772799002068217, 0.1647615404280894369, 0.1757036706920307445, 0.1866458009559719411, 0.2085300614838545563, 0.4016963878702066726, 0.4307237013227157574, 0.6771470142487683308, 1.000000000000000000 ),
 .UNSPECIFIED. ) ;
#10287=CARTESIAN_POINT ( 'NONE',  ( -1027.708477481198088, 65.70736702952430619, -99.57582448894528682 ) ) ;
#10296=CARTESIAN_POINT ( 'NONE',  ( -954.0832773815070595, 60.15510303592672869, -103.3307627799632513 ) ) ;
#10297=ADVANCED_FACE ( 'NONE', ( #7271, #11039 ), #8273, .F. ) ;
#10298=DIRECTION ( 'NONE',  ( 0.000000000000000000, -1.000000000000000000, -4.625929269271452387E-16 ) ) ;
#10308=CARTESIAN_POINT ( 'NONE',  ( -926.5908784743301112, 123.4113341959662762, -136.2353035311976441 ) ) ;
#10310=CARTESIAN_POINT ( 'NONE',  ( -1037.461794897084019, 110.6138330393709879, -107.9061927053326144 ) ) ;
#10317=CARTESIAN_POINT ( 'NONE',  ( -1031.476138302183244, 95.34216976508434982, -152.5758913445290830 ) ) ;
#10328=CARTESIAN_POINT ( 'NONE',  ( -853.4539021257704690, 72.48584973916007357, -154.8742214401226818 ) ) ;
#10346=CARTESIAN_POINT ( 'NONE',  ( -1038.595419435790973, 46.89684673038605922, -107.9061927053327850 ) ) ;
#10347=CARTESIAN_POINT ( 'NONE',  ( -818.8602300167407293, 79.32305858693317191, -104.8581405595893727 ) ) ;
#10349=CARTESIAN_POINT ( 'NONE',  ( -1025.976186494711783, 52.68972726728017619, -126.6442663926293193 ) ) ;
#10357=CARTESIAN_POINT ( 'NONE',  ( -1013.844210246976672, 57.79547239392030633, -107.9061927053327423 ) ) ;
#10367=CARTESIAN_POINT ( 'NONE',  ( -954.1708249681036023, 122.1961423320943680, -113.1262384684093263 ) ) ;
#10371=CARTESIAN_POINT ( 'NONE',  ( -1054.407929976941432, 113.5897173251036207, -118.7903414690678261 ) ) ;
#10378=CARTESIAN_POINT ( 'NONE',  ( -926.9570750291560444, 111.1083136274932031, -149.7857175106636021 ) ) ;
#10385=CARTESIAN_POINT ( 'NONE',  ( -1065.000000000002956, 76.10956187831469322, -154.2940595301282087 ) ) ;
#10386=PRODUCT_DEFINITION_FORMATION_WITH_SPECIFIED_SOURCE ( 'ANY', '', #6637, .NOT_KNOWN. ) ;
#10389=CARTESIAN_POINT ( 'NONE',  ( -819.8566349279940368, 81.72907896098652714, -154.3841807065155933 ) ) ;
#10392=CARTESIAN_POINT ( 'NONE',  ( -824.5038201930772175, 73.70910806073493404, -106.4800466717826595 ) ) ;
#10406=CARTESIAN_POINT ( 'NONE',  ( -1020.430183747026263, 74.13649791779302234, -96.78565065507955012 ) ) ;
#10407=DIRECTION ( 'NONE',  ( -1.000000000000000000, 1.262554838833776231E-16, 0.000000000000000000 ) ) ;
#10409=CARTESIAN_POINT ( 'NONE',  ( -1017.133222628203043, 54.07990892584120246, -130.5712005305404375 ) ) ;
#10410=EDGE_CURVE ( 'NONE', #9092, #5919, #2238, .T. ) ;
#10418=CARTESIAN_POINT ( 'NONE',  ( -853.9759289228104535, 31.63339360934237021, -107.9061927053328986 ) ) ;
#10432=CARTESIAN_POINT ( 'NONE',  ( -974.4564103291414767, 111.0951925441806480, -103.3307627799632371 ) ) ;
#10433=AXIS2_PLACEMENT_3D ( 'NONE', #12029, #7458, #2697 ) ;
#10443=CARTESIAN_POINT ( 'NONE',  ( -822.7482738817701602, 104.4536172844453148, -146.0307792196443017 ) ) ;
#10451=CARTESIAN_POINT ( 'NONE',  ( -903.6727718957008619, 110.0506089609179838, -149.7857175106632326 ) ) ;
#10452=CARTESIAN_POINT ( 'NONE',  ( -1010.947924043452645, 120.1731093567702828, -130.5712005305404375 ) ) ;
#10461=CARTESIAN_POINT ( 'NONE',  ( -818.9891295040824843, 77.37577012656028330, -105.2199448511381235 ) ) ;
#10462=CARTESIAN_POINT ( 'NONE',  ( -795.0000000000071623, 60.65002596136950075, -146.0307792196447565 ) ) ;
#10473=CARTESIAN_POINT ( 'NONE',  ( -1016.123300349496276, 74.17810748283143596, -96.78565065507957854 ) ) ;
#10474=CARTESIAN_POINT ( 'NONE',  ( -822.6918648528317135, 83.54617135776037173, -104.7406007859487715 ) ) ;
#10477=CARTESIAN_POINT ( 'NONE',  ( -818.8602280653290109, 79.32430977885860557, -144.5036099591918344 ) ) ;
#10482=CARTESIAN_POINT ( 'NONE',  ( -1062.493403002516516, 61.99900353997416147, -99.57582448894515892 ) ) ;
#10486=PRODUCT_DEFINITION_CONTEXT ( 'detailed design', #8448, 'design' ) ;
#10487=CARTESIAN_POINT ( 'NONE',  ( -954.1708249681036023, 122.1961423320943680, -113.1262384684093263 ) ) ;
#10495=CARTESIAN_POINT ( 'NONE',  ( -992.5689194452221500, 110.2481211102048491, -103.3307627799634218 ) ) ;
#10499=CARTESIAN_POINT ( 'NONE',  ( -954.0441199534441239, 124.9954171138387977, -122.7172756069788875 ) ) ;
#10503=CARTESIAN_POINT ( 'NONE',  ( -951.7027691703365235, 118.7449601027238799, -141.4553492942759192 ) ) ;
#10505=AXIS2_PLACEMENT_3D ( 'NONE', #5765, #7631, #10529 ) ;
#10510=CARTESIAN_POINT ( 'NONE',  ( -1022.719357623492101, 104.5170332807324769, -149.7857175106632610 ) ) ;
#10518=CARTESIAN_POINT ( 'NONE',  ( -819.3334343865132041, 76.46102376401721301, -105.4605772031392803 ) ) ;
#10519=CARTESIAN_POINT ( 'NONE',  ( -1025.000791045970800, 67.42844482392692385, -149.7857175106636305 ) ) ;
#10528=CARTESIAN_POINT ( 'NONE',  ( -1024.641217300039216, 73.20632742167531148, -96.78565065507991960 ) ) ;
#10529=DIRECTION ( 'NONE',  ( 4.236366511936864528E-16, -1.000000000000000000, -5.522905491341393153E-16 ) ) ;
#10537=CARTESIAN_POINT ( 'NONE',  ( -901.8967518049364571, 57.00804855647901093, -118.7903414690679540 ) ) ;
#10554=CARTESIAN_POINT ( 'NONE',  ( -952.4132309232843454, 101.5728619241205450, -96.78565065507918064 ) ) ;
#10560=CARTESIAN_POINT ( 'NONE',  ( -795.0000000000043201, 82.00000000000039790, -124.6807709998041105 ) ) ;
#10563=CARTESIAN_POINT ( 'NONE',  ( -1054.519145619990923, 111.4921997120091106, -136.2353035311978999 ) ) ;
#10571=CARTESIAN_POINT ( 'NONE',  ( -992.5689194452182846, 110.2481211102048491, -146.0307792196443870 ) ) ;
#10576=CARTESIAN_POINT ( 'NONE',  ( -828.8285638327243987, 78.67432280806596623, -144.4023295390031194 ) ) ;
#10577=CARTESIAN_POINT ( 'NONE',  ( -818.8285638327239440, 78.34163520102110567, -105.0153140909397393 ) ) ;
#10579=CARTESIAN_POINT ( 'NONE',  ( -1032.113539130925574, 67.34854938887519893, -152.5758913445294240 ) ) ;
#10590=CARTESIAN_POINT ( 'NONE',  ( -954.2862664537825594, 55.36536439393501041, -107.9061927053324439 ) ) ;
#10592=CARTESIAN_POINT ( 'NONE',  ( -1028.454949082223038, 53.01113643315406421, -136.2353035311987810 ) ) ;
#10597=CARTESIAN_POINT ( 'NONE',  ( -820.0628880458421008, 75.36885551798864924, -154.6770171190163126 ) ) ;
#10600=CARTESIAN_POINT ( 'NONE',  ( -1025.976186494711783, 52.68972726728017619, -122.7172756069792428 ) ) ;
#10606=CARTESIAN_POINT ( 'NONE',  ( -1011.418100375198719, 110.6663390795547599, -103.3307627799635782 ) ) ;
#10612=CARTESIAN_POINT ( 'NONE',  ( -1023.078931369429029, 98.73915068298381925, -96.78565065507928011 ) ) ;
#10616=CARTESIAN_POINT ( 'NONE',  ( -1060.756016675586807, 112.8516620848305934, -124.6807709998040821 ) ) ;
#10618=CARTESIAN_POINT ( 'NONE',  ( -852.8175266017511831, 121.6828083272127685, -124.6807709998041247 ) ) ;
#10621=CARTESIAN_POINT ( 'NONE',  ( -1046.095701327183860, 109.2451008237763546, -141.4553492942764308 ) ) ;
#10629=CARTESIAN_POINT ( 'NONE',  ( -828.8285638327247398, 78.67432280806576728, -154.5823979888776591 ) ) ;
#10630=CARTESIAN_POINT ( 'NONE',  ( -1013.875822516560447, 120.2710389253235519, -124.6807709998039257 ) ) ;
#10636=VECTOR ( 'NONE', #9515, 1000.000000000000000 ) ;
#10640=CARTESIAN_POINT ( 'NONE',  ( -975.9242088207953429, 48.36955882740826240, -146.0307792196450407 ) ) ;
#10641=CARTESIAN_POINT ( 'NONE',  ( -818.9567516184621354, 77.53771799247208207, -144.1773011583837558 ) ) ;
#10650=CARTESIAN_POINT ( 'NONE',  ( -976.0610374937461984, 42.74778062430068104, -107.9061927053324155 ) ) ;
#10661=CARTESIAN_POINT ( 'NONE',  ( -957.2086549536780922, 47.65337959301152893, -122.7172756069790012 ) ) ;
#10664=CARTESIAN_POINT ( 'NONE',  ( -992.5689194452221500, 110.2481211102048491, -103.3307627799634218 ) ) ;
#10670=CARTESIAN_POINT ( 'NONE',  ( -1031.632959140997855, 88.47632675500361188, -95.06748246948018277 ) ) ;
#10671=CARTESIAN_POINT ( 'NONE',  ( -951.4444194419925225, 124.5703232071644209, -130.5712005305403238 ) ) ;
#10674=CARTESIAN_POINT ( 'NONE',  ( -904.1919162299243453, 124.8346192645297918, -118.7903414690678119 ) ) ;
#10689=CARTESIAN_POINT ( 'NONE',  ( -903.8503739047791896, 115.2915043052427251, -146.0307792196441881 ) ) ;
#10695=CARTESIAN_POINT ( 'NONE',  ( -1060.756016675586807, 112.8516620848305934, -124.6807709998040821 ) ) ;
#10696=CARTESIAN_POINT ( 'NONE',  ( -927.8303129675907712, 79.95948428978974221, -152.5758913445291682 ) ) ;
#10697=CARTESIAN_POINT ( 'NONE',  ( -820.0477536417098463, 75.38653579115424463, -143.5572547269229062 ) ) ;
#10706=CARTESIAN_POINT ( 'NONE',  ( -1014.107508992743988, 52.59077491224116585, -130.5712005305404944 ) ) ;
#10707=CIRCLE ( 'NONE', #2414, 20.00000000000017053 ) ;
#10709=CARTESIAN_POINT ( 'NONE',  ( -1065.000000000004093, 52.00000000000021316, -122.7172756069792854 ) ) ;
#10716=CARTESIAN_POINT ( 'NONE',  ( -828.5739595068184826, 77.06538570633833274, -154.6543796050835624 ) ) ;
#10720=CARTESIAN_POINT ( 'NONE',  ( -1014.004070199759440, 54.58258344709550869, -113.1262384684095537 ) ) ;
#10724=CARTESIAN_POINT ( 'NONE',  ( -1046.676250823070177, 92.10743237175765330, -96.78565065507946485 ) ) ;
#10731=CARTESIAN_POINT ( 'NONE',  ( -1065.000000000005912, 82.00000000000039790, -94.48732055948609343 ) ) ;
#10733=CARTESIAN_POINT ( 'NONE',  ( -974.1288507787421622, 124.2142274477007078, -126.6442663926288787 ) ) ;
#10738=CARTESIAN_POINT ( 'NONE',  ( -1021.777026427247165, 118.8177985574657924, -118.7903414690675561 ) ) ;
#10748=CARTESIAN_POINT ( 'NONE',  ( -926.5138833012647410, 125.7648744980332225, -124.6807709998040394 ) ) ;
#10758=CARTESIAN_POINT ( 'NONE',  ( -1047.151245865163673, 77.61790247226322492, -154.8742214401233070 ) ) ;
#10763=SURFACE_STYLE_FILL_AREA ( #9535 ) ;
#10765=CARTESIAN_POINT ( 'NONE',  ( -956.9243412622475944, 54.10650223846812423, -141.4553492942761181 ) ) ;
#10770=CARTESIAN_POINT ( 'NONE',  ( -957.0819499390169085, 50.45265437475560333, -113.1262384684095537 ) ) ;
#10777=CARTESIAN_POINT ( 'NONE',  ( -828.8285638327248535, 78.34854159839228771, -154.6011532199805174 ) ) ;
#10781=CARTESIAN_POINT ( 'NONE',  ( -1017.133222628208614, 54.07990892584129483, -118.7903414690683519 ) ) ;
#10786=CARTESIAN_POINT ( 'NONE',  ( -1046.261572611724432, 104.4651992465225447, -103.3307627799636208 ) ) ;
#10793=CARTESIAN_POINT ( 'NONE',  ( -1011.935294340108044, 99.50314415908297860, -96.78565065507922327 ) ) ;
#10796=CARTESIAN_POINT ( 'NONE',  ( -1045.864486809339724, 115.5688325305733741, -124.6807709998043663 ) ) ;
#10804=CARTESIAN_POINT ( 'NONE',  ( -818.9960188511360002, 79.96793249489842026, -94.81477973375639579 ) ) ;
#10824=CARTESIAN_POINT ( 'NONE',  ( -817.4144546772251942, 30.82543593413060279, -136.2353035311987242 ) ) ;
#10830=CARTESIAN_POINT ( 'NONE',  ( -795.0000000000050022, 56.89504896194521422, -107.9061927053325860 ) ) ;
#10842=CARTESIAN_POINT ( 'NONE',  ( -1065.000000000005230, 87.89043812168627312, -95.06748246948058068 ) ) ;
#10851=CARTESIAN_POINT ( 'NONE',  ( -1062.096538105501168, 73.81465972843167833, -95.06748246948046699 ) ) ;
#10854=CARTESIAN_POINT ( 'NONE',  ( -795.0000000000040927, 111.6133447792292088, -130.5712005305403522 ) ) ;
#10859=CARTESIAN_POINT ( 'NONE',  ( -820.0616184920847900, 81.97828950705842033, -95.00646471220841249 ) ) ;
#10862=CARTESIAN_POINT ( 'NONE',  ( -795.0000000000046612, 112.0000000000007532, -122.7172756069791717 ) ) ;
#10871=CARTESIAN_POINT ( 'NONE',  ( -975.3893330992545998, 71.12659035875127245, -154.2940595301280950 ) ) ;
#10872=CARTESIAN_POINT ( 'NONE',  ( -826.9024563477421452, 74.71743289348884787, -143.3087845970618162 ) ) ;
#10876=CARTESIAN_POINT ( 'NONE',  ( -826.0494213903788250, 74.18265558624132439, -94.69403889809616715 ) ) ;
#10878=ORIENTED_EDGE ( 'NONE', *, *, #5649, .F. ) ;
#10879=CARTESIAN_POINT ( 'NONE',  ( -853.9759289228051102, 31.63339360934212152, -141.4553492942759192 ) ) ;
#10888=CARTESIAN_POINT ( 'NONE',  ( -828.1603582063153226, 81.17680912107698532, -94.97408237440919265 ) ) ;
#10899=CARTESIAN_POINT ( 'NONE',  ( -903.0443340174317655, 90.92133391050421665, -94.48732055948569553 ) ) ;
#10904=DIRECTION ( 'NONE',  ( 0.000000000000000000, 0.000000000000000000, 1.000000000000000000 ) ) ;
#10905=ORIENTED_EDGE ( 'NONE', *, *, #948, .T. ) ;
#10912=CARTESIAN_POINT ( 'NONE',  ( -1056.430032577878137, 71.19035303699463668, -95.06748246948046699 ) ) ;
#10917=CARTESIAN_POINT ( 'NONE',  ( -1013.901471336336158, 119.8325901201402814, -118.7903414690677835 ) ) ;
#10926=CARTESIAN_POINT ( 'NONE',  ( -991.5701548301636876, 122.8678427087060214, -124.6807709998040536 ) ) ;
#10950=CARTESIAN_POINT ( 'NONE',  ( -1020.755281158171670, 68.40999151392655619, -149.7857175106638010 ) ) ;
#10959=ORIENTED_EDGE ( 'NONE', *, *, #7525, .F. ) ;
#10962=CARTESIAN_POINT ( 'NONE',  ( -1014.132585063772808, 52.13780504951625261, -126.6442663926290777 ) ) ;
#10966=CARTESIAN_POINT ( 'NONE',  ( -853.4539021257702416, 72.48584973915980356, -94.48732055948642028 ) ) ;
#10973=ORIENTED_EDGE ( 'NONE', *, *, #3438, .F. ) ;
#10975=CARTESIAN_POINT ( 'NONE',  ( -955.9230626098324137, 78.80814421416175719, -95.06748246948052383 ) ) ;
#10989=CARTESIAN_POINT ( 'NONE',  ( -951.4444194419894529, 124.5703232071642503, -118.7903414690678829 ) ) ;
#11000=CARTESIAN_POINT ( 'NONE',  ( -824.4897464405680694, 73.71539350114069578, -142.8842219741777342 ) ) ;
#11009=CARTESIAN_POINT ( 'NONE',  ( -1032.391769651406321, 55.42093464310143247, -146.0307792196449839 ) ) ;
#11018=EDGE_LOOP ( 'NONE', ( #3477, #8618, #7253, #8693 ) ) ;
#11021=CARTESIAN_POINT ( 'NONE',  ( -817.1493800258450619, 27.50875274330017461, -126.6442663926291630 ) ) ;
#11028=CARTESIAN_POINT ( 'NONE',  ( -1037.899050076301137, 86.18944477603540122, -95.06748246948046699 ) ) ;
#11035=CARTESIAN_POINT ( 'NONE',  ( -821.6111871957904214, 83.16774079293004718, -154.1944187633729939 ) ) ;
#11036=CARTESIAN_POINT ( 'NONE',  ( -956.2104666674714508, 71.56905446038054208, -96.78565065507946485 ) ) ;
#11039=FACE_BOUND ( 'NONE', #8890, .T. ) ;
#11041=FACE_OUTER_BOUND ( 'NONE', #11209, .T. ) ;
#11049=CARTESIAN_POINT ( 'NONE',  ( -819.1467617552298179, 76.91148745156876032, -154.6757676722768906 ) ) ;
#11052=CARTESIAN_POINT ( 'NONE',  ( -1024.691966601154036, 118.8493250655916142, -122.7172756069790580 ) ) ;
#11059=CARTESIAN_POINT ( 'NONE',  ( -1013.875822516560447, 120.2710389253235519, -124.6807709998039257 ) ) ;
#11063=CARTESIAN_POINT ( 'NONE',  ( -821.6815100408632588, 89.78153722040215712, -152.5758913445288840 ) ) ;
#11074=CARTESIAN_POINT ( 'NONE',  ( -1062.096538105497302, 73.81465972843197676, -154.2940595301284930 ) ) ;
#11091=CARTESIAN_POINT ( 'NONE',  ( -927.2951026182247460, 99.13268410970638911, -95.06748246948001224 ) ) ;
#11094=CARTESIAN_POINT ( 'NONE',  ( -795.0000000000038654, 109.8950841424301359, -136.2353035311980136 ) ) ;
#11095=CARTESIAN_POINT ( 'NONE',  ( -823.1761409384637318, 83.64233031452228317, -144.6133277457492170 ) ) ;
#11101=CARTESIAN_POINT ( 'NONE',  ( -1056.743458481016432, 64.45745743522633120, -96.78565065507969223 ) ) ;
#11103=DIRECTION ( 'NONE',  ( 1.000000000000000000, -1.262554838833776231E-16, 0.000000000000000000 ) ) ;
#11115=CARTESIAN_POINT ( 'NONE',  ( -904.1167769183923610, 122.8348148996190758, -136.2353035311977862 ) ) ;
#11117=CARTESIAN_POINT ( 'NONE',  ( -926.5289067496665893, 125.3297071905304421, -118.7903414690680535 ) ) ;
#11120=LINE ( 'NONE', #477, #3719 ) ;
#11127=CARTESIAN_POINT ( 'NONE',  ( -1014.911393615049064, 99.73439156315002663, -152.5758913445290261 ) ) ;
#11131=CARTESIAN_POINT ( 'NONE',  ( -974.7984820115178763, 96.63273410478066694, -152.5758913445288272 ) ) ;
#11138=CARTESIAN_POINT ( 'NONE',  ( -1065.000000000007958, 70.44548139156172795, -152.5758913445293388 ) ) ;
#11158=CARTESIAN_POINT ( 'NONE',  ( -1047.626240907246483, 63.12837257276869707, -96.78565065507969223 ) ) ;
#11170=CARTESIAN_POINT ( 'NONE',  ( -853.7969483066802923, 45.36294356226295577, -99.57582448894520155 ) ) ;
#11187=CARTESIAN_POINT ( 'NONE',  ( -904.1167769183953169, 122.8348148996191611, -113.1262384684093263 ) ) ;
#11196=APPLICATION_CONTEXT ( 'automotive_design' ) ;
#11199=CARTESIAN_POINT ( 'NONE',  ( -994.1998135634695473, 88.30642396300672203, -154.2940595301282656 ) ) ;
#11207=CARTESIAN_POINT ( 'NONE',  ( -1038.028607166442953, 78.75533988487831039, -154.8742214401230797 ) ) ;
#11209=EDGE_LOOP ( 'NONE', ( #5148, #5917, #5749, #10973 ) ) ;
#11213=CARTESIAN_POINT ( 'NONE',  ( -828.1717276517556456, 76.17609097696481513, -105.5454165443659491 ) ) ;
#11223=MECHANICAL_DESIGN_GEOMETRIC_PRESENTATION_REPRESENTATION('',(#751),#5877);
#11226=CARTESIAN_POINT ( 'NONE',  ( -1021.293373424897709, 59.24127555818995461, -107.9061927053327281 ) ) ;
#11238=CARTESIAN_POINT ( 'NONE',  ( -1057.036663358159558, 58.23757105449750071, -99.57582448894497418 ) ) ;
#11239=CARTESIAN_POINT ( 'NONE',  ( -1065.000000000006366, 82.00000000000036948, -124.6807709998044231 ) ) ;
#11252=CARTESIAN_POINT ( 'NONE',  ( -1037.550865396562358, 105.7975851359348241, -103.3307627799636350 ) ) ;
#11261=CARTESIAN_POINT ( 'NONE',  ( -1037.899050076299318, 86.18944477603574228, -154.2940595301282656 ) ) ;
#11266=CARTESIAN_POINT ( 'NONE',  ( -927.4753839990684128, 92.66010094724849466, -154.8742214401223691 ) ) ;
#11269=VERTEX_POINT ( 'NONE', #439 ) ;
#11271=CARTESIAN_POINT ( 'NONE',  ( -1032.503061859593117, 50.81309391744441228, -141.4553492942758908 ) ) ;
#11280=CARTESIAN_POINT ( 'NONE',  ( -1027.375436305349467, 71.63039521860197567, -96.78565065507956433 ) ) ;
#11281=CARTESIAN_POINT ( 'NONE',  ( -819.8468830326183934, 81.71630402067619059, -104.6809196082603961 ) ) ;
#11282=CARTESIAN_POINT ( 'NONE',  ( -1062.996098538724254, 47.98024286075312261, -130.5712005305402101 ) ) ;
#11288=CARTESIAN_POINT ( 'NONE',  ( -1025.595947590972401, 58.17469240935120922, -107.9061927053327707 ) ) ;
#11298=CARTESIAN_POINT ( 'NONE',  ( -1065.000000000008868, 103.3499740386314016, -103.3307627799635924 ) ) ;
#11304=CARTESIAN_POINT ( 'NONE',  ( -1054.380968608932108, 114.0683136310379524, -122.7172756069792570 ) ) ;
#11306=CARTESIAN_POINT ( 'NONE',  ( -926.5138833012647410, 125.7648744980332225, -124.6807709998040394 ) ) ;
#11309=CARTESIAN_POINT ( 'NONE',  ( -1019.017691546887363, 99.44610047464912839, -152.5758913445291967 ) ) ;
#11317=CARTESIAN_POINT ( 'NONE',  ( -853.6888141844391384, 53.84495383942815039, -152.5758913445293103 ) ) ;
#11324=CARTESIAN_POINT ( 'NONE',  ( -828.3259789886610633, 76.46577308275233520, -105.4592182070451543 ) ) ;
#11326=CARTESIAN_POINT ( 'NONE',  ( -1048.206790403134164, 45.99070412075050740, -141.4553492942756918 ) ) ;
#11335=CARTESIAN_POINT ( 'NONE',  ( -1047.844889418690855, 56.55730854968127375, -99.57582448894520155 ) ) ;
#11336=CARTESIAN_POINT ( 'NONE',  ( -824.1545993022754146, 83.67440335600112178, -104.7509849144500578 ) ) ;
#11337=CARTESIAN_POINT ( 'NONE',  ( -1025.943122242211757, 53.12767954719351593, -130.5712005305404375 ) ) ;
#11347=CARTESIAN_POINT ( 'NONE',  ( -853.8938961404153360, 37.86297855175766358, -103.3307627799636776 ) ) ;
#11361=CARTESIAN_POINT ( 'NONE',  ( -1014.382386707157252, 110.5980896718282196, -103.3307627799636350 ) ) ;
#11365=CARTESIAN_POINT ( 'NONE',  ( -1065.000000000007731, 112.0000000000007105, -122.7172756069790438 ) ) ;
#11371=CARTESIAN_POINT ( 'NONE',  ( -903.6727718957008619, 110.0506089609179838, -149.7857175106632326 ) ) ;
#11387=CARTESIAN_POINT ( 'NONE',  ( -996.5513353153702383, 56.29506814688406990, -149.7857175106634600 ) ) ;
#11395=CARTESIAN_POINT ( 'NONE',  ( -997.7839878466141954, 40.27522178589210711, -136.2353035311988378 ) ) ;
#11399=CARTESIAN_POINT ( 'NONE',  ( -1021.046747802643722, 63.38047825189596551, -103.3307627799639761 ) ) ;
#11400=CARTESIAN_POINT ( 'NONE',  ( -818.8285638327243987, 79.00074005404812283, -104.9041682110414371 ) ) ;
#11409=CARTESIAN_POINT ( 'NONE',  ( -1038.401083800584274, 57.54275223462379074, -99.57582448894500260 ) ) ;
#11411=B_SPLINE_CURVE_WITH_KNOTS ( 'NONE', 3,
 ( #7510, #11400, #10347, #2937, #6701, #11463, #8688, #11281, #6583, #1891, #16, #5653, #1149, #6823, #195, #2132, #10474, #8507, #138, #11336, #12213, #9606, #9427, #3980, #8455, #3921, #3793, #2009, #9543, #7749, #963, #5890, #7690, #2994, #7567, #2877, #6755, #4791 ),
 .UNSPECIFIED., .F., .F.,
 ( 4, 2, 2, 2, 2, 2, 2, 2, 2, 2, 2, 2, 2, 2, 2, 2, 2, 2, 4 ),
 ( 0.000000000000000000, 0.0009791294386042174221, 0.001958258877208434844, 0.002937388315812651616, 0.003916517754416869689, 0.004895647193021087328, 0.005874776631625303232, 0.006364341350927419858, 0.006853906070229536483, 0.007833035508834094995, 0.008812164947438654375, 0.009791294386043212020, 0.01077042382464777140, 0.01174955326325232731, 0.01272868270185688495, 0.01370781214046144433, 0.01468694157906600198, 0.01517650629836831376, 0.01566607101767062554 ),
 .UNSPECIFIED. ) ;
#11413=CARTESIAN_POINT ( 'NONE',  ( -1014.170783943992433, 114.7803637426472534, -107.9061927053325292 ) ) ;
#11421=CARTESIAN_POINT ( 'NONE',  ( -853.0139081111171890, 107.1087209265617020, -103.3307627799635355 ) ) ;
#11422=AXIS2_PLACEMENT_3D ( 'NONE', #2947, #1837, #9438 ) ;
#11427=CARTESIAN_POINT ( 'NONE',  ( -1024.691966601152672, 118.8493250655916142, -124.6807709998039400 ) ) ;
#11432=CARTESIAN_POINT ( 'NONE',  ( -954.5323978148076094, 113.6695689568733911, -146.0307792196442165 ) ) ;
#11438=CARTESIAN_POINT ( 'NONE',  ( -954.5323978148076094, 113.6695689568733911, -146.0307792196442165 ) ) ;
#11449=CARTESIAN_POINT ( 'NONE',  ( -1032.260242496265846, 61.00429285198246987, -149.7857175106635452 ) ) ;
#11456=CARTESIAN_POINT ( 'NONE',  ( -976.2351830774960035, 35.86345807843989775, -130.5712005305402101 ) ) ;
#11462=CARTESIAN_POINT ( 'NONE',  ( -1013.637332661006667, 62.09754518945625534, -103.3307627799637913 ) ) ;
#11463=CARTESIAN_POINT ( 'NONE',  ( -819.3307005430699519, 80.88259174529733286, -104.7097040407758328 ) ) ;
#11474=CARTESIAN_POINT ( 'NONE',  ( -928.3598895237944362, 61.90886769853011629, -113.1262384684093831 ) ) ;
#11485=CARTESIAN_POINT ( 'NONE',  ( -1065.000000000002956, 98.77454568802522772, -99.57582448894488891 ) ) ;
#11487=CARTESIAN_POINT ( 'NONE',  ( -1045.967528061855091, 112.8272211019271225, -136.2353035311980705 ) ) ;
#11494=CARTESIAN_POINT ( 'NONE',  ( -1022.396981161619806, 109.5926079579672603, -146.0307792196444154 ) ) ;
#11500=CARTESIAN_POINT ( 'NONE',  ( -1018.692594135740137, 105.1726068785159214, -149.7857175106633747 ) ) ;
#11508=CARTESIAN_POINT ( 'NONE',  ( -1065.000000000007958, 70.44548139156172795, -152.5758913445293388 ) ) ;
#11518=CARTESIAN_POINT ( 'NONE',  ( -901.8967518049312275, 57.00804855647886171, -130.5712005305400965 ) ) ;
#11522=CARTESIAN_POINT ( 'NONE',  ( -956.9243412622536198, 54.10650223846825924, -107.9061927053324439 ) ) ;
#11523=DIRECTION ( 'NONE',  ( 0.000000000000000000, -1.000000000000000000, -4.625929269271452387E-16 ) ) ;
#11524=CARTESIAN_POINT ( 'NONE',  ( -1062.923339974281134, 49.86928741160674150, -136.2353035311989515 ) ) ;
#11533=CARTESIAN_POINT ( 'NONE',  ( -795.0000000000061391, 52.38665522077228331, -118.7903414690680250 ) ) ;
#11540=PRODUCT_DEFINITION ( 'UNKNOWN', '', #10386, #10486 ) ;
#11541=CARTESIAN_POINT ( 'NONE',  ( -954.3284336448667773, 118.5422944683823800, -107.9061927053323302 ) ) ;
#11549=CARTESIAN_POINT ( 'NONE',  ( -1012.226803665789134, 93.06815595962675047, -95.06748246948018277 ) ) ;
#11559=CARTESIAN_POINT ( 'NONE',  ( -823.1749794181308744, 110.1592441374104112, -141.4553492942763171 ) ) ;
#11566=CARTESIAN_POINT ( 'NONE',  ( -1045.864486809339724, 115.5688325305733741, -124.6807709998043663 ) ) ;
#11573=CARTESIAN_POINT ( 'NONE',  ( -976.0610374937396045, 42.74778062430040393, -141.4553492942756634 ) ) ;
#11580=AXIS2_PLACEMENT_3D ( 'NONE', #12043, #4377, #1958 ) ;
#11585=CARTESIAN_POINT ( 'NONE',  ( -828.8285638327245124, 78.67432280806571043, -264.6807709998050200 ) ) ;
#11587=CARTESIAN_POINT ( 'NONE',  ( -1048.334963668458158, 42.40858384259915681, -113.1262384684096105 ) ) ;
#11589=CARTESIAN_POINT ( 'NONE',  ( -957.1839320239870403, 48.17551948191491817, -130.5712005305400112 ) ) ;
#11598=CARTESIAN_POINT ( 'NONE',  ( -998.0431609429222135, 37.14019503514177956, -122.7172756069792854 ) ) ;
#11603=CARTESIAN_POINT ( 'NONE',  ( -1046.457602311629898, 98.67849639484570901, -99.57582448894517313 ) ) ;
#11613=CARTESIAN_POINT ( 'NONE',  ( -1055.469533842434430, 91.91071092603658599, -96.78565065507918064 ) ) ;
#11615=CARTESIAN_POINT ( 'NONE',  ( -1037.392967692951970, 114.2240391150264998, -136.2353035311982126 ) ) ;
#11616=DIRECTION ( 'NONE',  ( 1.000000000000000000, -1.262554838833776231E-16, 0.000000000000000000 ) ) ;
#11618=CARTESIAN_POINT ( 'NONE',  ( -926.5289067496665893, 125.3297071905304421, -118.7903414690680535 ) ) ;
#11632=CARTESIAN_POINT ( 'NONE',  ( -1011.211222789229396, 114.9684118750914621, -141.4553492942763455 ) ) ;
#11639=CARTESIAN_POINT ( 'NONE',  ( -795.0000000000011369, 65.22545431197602284, -149.7857175106635452 ) ) ;
#11640=CARTESIAN_POINT ( 'NONE',  ( -819.4840074578181657, 76.17856360854504771, -143.8168744253326565 ) ) ;
#11647=CARTESIAN_POINT ( 'NONE',  ( -1025.806732200646138, 55.05754055295012961, -113.1262384684095537 ) ) ;
#11653=CARTESIAN_POINT ( 'NONE',  ( -826.0420070959999066, 74.18794025998390396, -154.6674632209163178 ) ) ;
#11657=CARTESIAN_POINT ( 'NONE',  ( -1063.013736978594579, 47.55218547899811199, -126.6442663926291914 ) ) ;
#11662=CARTESIAN_POINT ( 'NONE',  ( -822.2439855206088168, 97.57287547056382948, -99.57582448894494576 ) ) ;
#11670=CARTESIAN_POINT ( 'NONE',  ( -903.2629211055218548, 97.63080833215146015, -95.06748246947979908 ) ) ;
#11673=CARTESIAN_POINT ( 'NONE',  ( -1030.944970944897250, 117.4714819019839354, -130.5712005305406649 ) ) ;
#11674=CARTESIAN_POINT ( 'NONE',  ( -795.0000000000035243, 112.0000000000008953, -126.6442663926293477 ) ) ;
#11682=CARTESIAN_POINT ( 'NONE',  ( -951.4198147059589701, 125.0824040815807194, -124.6807709998040252 ) ) ;
#11683=B_SPLINE_SURFACE_WITH_KNOTS ( 'NONE', 3, 3, ( 
 ( #8220, #9939, #2639, #11917, #12112, #2457, #6176, #12044, #1474, #3623, #11981, #10926, #3436, #5291, #10189, #1534, #6236, #5234, #9068, #1590 ),
 ( #668, #2516, #5415, #10122, #603, #1655, #11052, #6292, #732, #10002, #9005, #1729, #4378, #5487, #10061, #8151, #538, #3372, #4574, #10862 ),
 ( #9196, #8094, #3497, #7223, #9261, #5353, #4507, #803, #6417, #7286, #8287, #3555, #9129, #7162, #10989, #11117, #4443, #2397, #4320, #2577 ),
 ( #6349, #7345, #104, #5552, #8417, #9389, #12237, #2836, #928, #2028, #6481, #4701, #6603, #10367, #7531, #1908, #11187, #9568, #5785, #38 ),
 ( #8475, #1110, #7590, #3880, #10310, #5673, #3757, #2957, #868, #4638, #10255, #9506, #2709, #155, #4861, #3816, #12180, #3696, #8647, #1850 ),
 ( #11298, #7410, #7472, #985, #11252, #2777, #6662, #6540, #8526, #11361, #2898, #10495, #10432, #1975, #5731, #1051, #7651, #11421, #6720, #7709 ),
 ( #11485, #2151, #2330, #3018, #8873, #6779, #6962, #3074, #11727, #9623, #4069, #3129, #3242, #7022, #4003, #5850, #6846, #2269, #7836, #397 ),
 ( #6101, #8819, #11613, #9684, #9871, #4126, #1343, #10612, #6902, #5918, #10793, #1171, #4180, #4925, #10554, #2206, #8704, #5975, #9742, #6038 ),
 ( #2096, #219, #345, #7772, #1400, #10670, #5164, #8924, #3941, #1287, #11549, #3185, #1224, #4981, #8763, #7901, #11670, #282, #9804, #5041 ),
 ( #10731, #5106, #7959, #5469, #6280, #10050, #11787, #4492, #1518, #10175, #4309, #8020, #1641, #7083, #1710, #1581, #523, #5280, #7146, #12028 ),
 ( #8080, #10851, #10912, #3420, #454, #2503, #4367, #7269, #3484, #2442, #653, #10109, #3361, #10975, #6225, #8270, #2386, #717, #6158, #9924 ),
 ( #5342, #8992, #11101, #9989, #9116, #2625, #6403, #4430, #6336, #5219, #8206, #4249, #11849, #11036, #2565, #9055, #593, #8136, #11902, #5720 ),
 ( #2763, #10482, #11238, #3746, #11409, #4744, #9246, #4623, #4558, #12166, #6650, #8334, #3868, #2946, #91, #9436, #6709, #11170, #1775, #919 ),
 ( #2695, #788, #9311, #6467, #12221, #4688, #6527, #7455, #12098, #5537, #8462, #3607, #7398, #3680, #10296, #10240, #853, #11347, #8402, #2017 ),
 ( #1899, #1836, #5599, #7640, #9376, #8515, #7518, #11288, #2821, #6589, #10357, #5662, #28, #972, #3802, #7575, #2889, #10418, #1960, #9493 ),
 ( #1035, #4799, #8569, #5965, #9551, #6764, #1097, #3992, #4170, #4851, #10720, #8631, #8808, #4911, #1331, #11474, #5905, #4972, #5091, #8863 ),
 ( #7701, #8696, #4116, #9676, #2256, #9613, #6892, #5775, #146, #10781, #3230, #6028, #265, #3005, #3931, #5838, #10537, #8752, #1214, #11533 ),
 ( #2084, #1158, #4057, #207, #7760, #3062, #6831, #10600, #2140, #7888, #7824, #11598, #388, #10661, #3116, #2197, #7944, #9733, #5031, #1272 ),
 ( #329, #11657, #3176, #6952, #9791, #11717, #7009, #9909, #437, #5387, #10962, #506, #2490, #6266, #10037, #1567, #8183, #6086, #11021, #4227 ),
 ( #702, #10094, #1628, #9165, #4477, #12012, #10157, #1082, #7741, #4957, #10706, #2242, #11456, #9536, #2062, #8794, #11518, #313, #2988, #251 ),
 ( #2004, #378, #7627, #4101, #4040, #1142, #7873, #3164, #3044, #6694, #4893, #11395, #8617, #3914, #190, #6010, #425, #9086, #10824, #5252 ),
 ( #1494, #10022, #6995, #6193, #1552, #8171, #7180, #2413, #8111, #2365, #494, #7930, #625, #10765, #9898, #5374, #6131, #10879, #6313, #11874 ),
 ( #11764, #11704, #7052, #5316, #3219, #11009, #10081, #7243, #4341, #1612, #6071, #8898, #8053, #2301, #1434, #9150, #5192, #9961, #4157, #3390 ),
 ( #3277, #9836, #8964, #4397, #1375, #2538, #5138, #4215, #10950, #7993, #4283, #11820, #3339, #9024, #7117, #561, #2478, #6255, #11939, #3457 ),
 ( #11138, #4465, #5437, #12135, #3519, #7311, #3576, #10210, #10144, #12002, #2795, #8242, #5687, #7548, #5570, #1679, #9217, #11317, #7367, #12197 ),
 ( #10385, #11074, #1748, #756, #4533, #3715, #8309, #2600, #12066, #6372, #3775, #5510, #2665, #2732, #6439, #9285, #823, #887, #4596, #8370 ),
 ( #3648, #2858, #7427, #5633, #11207, #7492, #6500, #8491, #10274, #1808, #9345, #12239, #6622, #4658, #8434, #11266, #6563, #10328, #9407, #1869 ),
 ( #689, #943, #4715, #1926, #11261, #2724, #8303, #8428, #6494, #6433, #1605, #1672, #6306, #10074, #2532, #4526, #3641, #9211, #1862, #747 ),
 ( #4711, #5626, #5564, #12193, #9144, #9339, #3708, #9402, #8487, #684, #4457, #12058, #11131, #8236, #11996, #7303, #3570, #7362, #2659, #10203 ),
 ( #754, #2731, #2664, #59, #2794, #11686, #7792, #10510, #11500, #3957, #1305, #1127, #5806, #9522, #7725, #1188, #10451, #237, #2110, #5000 ),
 ( #3028, #9705, #5935, #5867, #302, #2044, #4824, #5058, #6798, #7919, #9643, #10571, #8600, #11438, #3205, #1989, #10689, #1244, #7669, #3095 ),
 ( #119, #6735, #1067, #5747, #4943, #3896, #4022, #8719, #4088, #7857, #11632, #9586, #3150, #2225, #5991, #9131, #7593, #4983, #2901, #6849 ),
 ( #7840, #5734, #158, #11487, #11615, #3133, #107, #9508, #5786, #2155, #3943, #8765, #3883, #4926, #41, #6663, #5044, #9744, #284, #8705 ),
 ( #1227, #4006, #7710, #1053, #9569, #3818, #4811, #8583, #3019, #2098, #7653, #4072, #9625, #220, #10671, #6906, #2208, #5976, #1289, #10854 ),
 ( #10052, #2388, #4183, #8084, #7024, #7904, #6964, #8995, #526, #3188, #7148, #11905, #10733, #2271, #3424, #5221, #7961, #6040, #1346, #11674 ),
 ( #9873, #9807, #6160, #10796, #5166, #1403, #4311, #347, #5109, #4128, #2332, #7210, #8876, #1521, #399, #11851, #11730, #8140, #3245, #8927 ) ),
 .UNSPECIFIED., .T., .F., .F.,
 ( 4, 1, 1, 1, 1, 1, 1, 1, 1, 1, 1, 1, 1, 1, 1, 1, 2, 1, 1, 1, 1, 1, 1, 1, 1, 1, 1, 1, 1, 1, 1, 1, 4 ),
 ( 4, 1, 1, 1, 2, 1, 1, 1, 2, 2, 2, 2, 4 ),
 ( 0.000000000000000000, 0.03125000000000000000, 0.06250000000000000000, 0.09375000000000000000, 0.1250000000000000000, 0.1562500000000000000, 0.1875000000000000000, 0.2187500000000000000, 0.2500000000000000000, 0.2812500000000000000, 0.3125000000000000000, 0.3437500000000000000, 0.3750000000000000000, 0.4062500000000000000, 0.4375000000000000000, 0.4687500000000000000, 0.5000000000000000000, 0.5312500000000000000, 0.5625000000000000000, 0.5937500000000000000, 0.6250000000000000000, 0.6562500000000000000, 0.6875000000000000000, 0.7187500000000000000, 0.7500000000000000000, 0.7812500000000000000, 0.8125000000000000000, 0.8437500000000000000, 0.8750000000000000000, 0.9062500000000000000, 0.9375000000000000000, 0.9687500000000000000, 1.000000000000000000 ),
 ( 0.000000000000000000, 0.04762575996673557022, 0.07143863995010346635, 0.09525151993347125146, 0.1428772799002068217, 0.1647615404280894369, 0.1757036706920307445, 0.1866458009559719411, 0.2085300614838545563, 0.4016963878702066726, 0.4307237013227157574, 0.6771470142487683308, 1.000000000000000000 ),
 .UNSPECIFIED. ) ;
#11686=CARTESIAN_POINT ( 'NONE',  ( -1031.329434936838197, 101.6864263019769083, -149.7857175106636305 ) ) ;
#11694=CARTESIAN_POINT ( 'NONE',  ( -853.6888141844391384, 53.84495383942815039, -152.5758913445293103 ) ) ;
#11695=CARTESIAN_POINT ( 'NONE',  ( -820.5015944640223324, 74.92794535928011612, -143.3902763353424348 ) ) ;
#11700=CARTESIAN_POINT ( 'NONE',  ( -827.1370682460163835, 74.91132569719390233, -94.68188112044103377 ) ) ;
#11704=CARTESIAN_POINT ( 'NONE',  ( -1062.665377791219498, 57.01990411978283646, -146.0307792196448702 ) ) ;
#11709=CARTESIAN_POINT ( 'NONE',  ( -997.4616017999825317, 44.34671234275855767, -107.9061927053325007 ) ) ;
#11711=CARTESIAN_POINT ( 'NONE',  ( -828.6680473269018421, 79.97282626266093075, -94.86685776557048655 ) ) ;
#11714=CARTESIAN_POINT ( 'NONE',  ( -821.3231414384459868, 74.33484277641235849, -154.6590659353650494 ) ) ;
#11717=CARTESIAN_POINT ( 'NONE',  ( -1032.658196452833636, 44.72920460984212809, -126.6442663926291914 ) ) ;
#11721=CARTESIAN_POINT ( 'NONE',  ( -1014.911393615048723, 99.73439156314999821, -96.78565065507932275 ) ) ;
#11727=CARTESIAN_POINT ( 'NONE',  ( -1018.692594135739682, 105.1726068785156656, -99.57582448894508786 ) ) ;
#11729=CARTESIAN_POINT ( 'NONE',  ( -974.1454360724337675, 123.6012932931491690, -130.5712005305403238 ) ) ;
#11730=CARTESIAN_POINT ( 'NONE',  ( -904.2101318205999405, 125.2895275102983419, -124.6807709998041531 ) ) ;
#11736=CARTESIAN_POINT ( 'NONE',  ( -1024.848917040348397, 116.4131098345821442, -113.1262384684097242 ) ) ;
#11741=CARTESIAN_POINT ( 'NONE',  ( -1021.637154595298057, 53.81063926482157456, -124.6807709998041958 ) ) ;
#11751=EDGE_LOOP ( 'NONE', ( #5022, #8743, #5083, #9349 ) ) ;
#11757=CARTESIAN_POINT ( 'NONE',  ( -819.2376510598713821, 55.50059629688480811, -152.5758913445292535 ) ) ;
#11764=CARTESIAN_POINT ( 'NONE',  ( -1065.000000000007731, 60.65002596136951496, -146.0307792196448986 ) ) ;
#11768=CARTESIAN_POINT ( 'NONE',  ( -1021.483947769352199, 56.15424078096101113, -113.1262384684096105 ) ) ;
#11770=CARTESIAN_POINT ( 'NONE',  ( -826.0438798663770967, 83.15978422364159428, -95.19800250875974257 ) ) ;
#11780=CARTESIAN_POINT ( 'NONE',  ( -853.2189900670988436, 91.12674563889150647, -96.78565065507912379 ) ) ;
#11785=ORIENTED_EDGE ( 'NONE', *, *, #10410, .T. ) ;
#11787=CARTESIAN_POINT ( 'NONE',  ( -1026.651933061283898, 84.71212313386838844, -94.48732055948616448 ) ) ;
#11798=CARTESIAN_POINT ( 'NONE',  ( -819.1470717756643580, 80.43796722965394963, -94.85155950616754694 ) ) ;
#11802=CARTESIAN_POINT ( 'NONE',  ( -795.0000000000047748, 112.0000000000007532, -124.6807709998042384 ) ) ;
#11812=CARTESIAN_POINT ( 'NONE',  ( -1056.430032577873362, 71.19035303699479300, -154.2940595301283793 ) ) ;
#11813=CARTESIAN_POINT ( 'NONE',  ( -821.1548363108421427, 74.44610204637938011, -143.1996371447164904 ) ) ;
#11820=CARTESIAN_POINT ( 'NONE',  ( -996.5513353153702383, 56.29506814688406990, -149.7857175106634600 ) ) ;
#11829=CARTESIAN_POINT ( 'NONE',  ( -827.8052707278029629, 81.72255078513846627, -95.02959508169305991 ) ) ;
#11840=CARTESIAN_POINT ( 'NONE',  ( -903.6727718956999524, 110.0506089609176712, -99.57582448894470417 ) ) ;
#11848=CARTESIAN_POINT ( 'NONE',  ( -828.1698196941869128, 81.17660424754099324, -154.3879017162145146 ) ) ;
#11849=CARTESIAN_POINT ( 'NONE',  ( -975.5821371384171243, 62.83201726680821508, -96.78565065507949328 ) ) ;
#11851=CARTESIAN_POINT ( 'NONE',  ( -926.5138833012647410, 125.7648744980332225, -124.6807709998040394 ) ) ;
#11863=EDGE_LOOP ( 'NONE', ( #11924, #10079 ) ) ;
#11870=CARTESIAN_POINT ( 'NONE',  ( -824.1630149179034106, 73.67461580146778033, -94.71311452716244617 ) ) ;
#11874=CARTESIAN_POINT ( 'NONE',  ( -795.0000000000002274, 56.89504896194490868, -141.4553492942756350 ) ) ;
#11891=CARTESIAN_POINT ( 'NONE',  ( -975.1903095749676140, 79.73237568579435219, -94.48732055948607922 ) ) ;
#11898=( NAMED_UNIT ( * ) PLANE_ANGLE_UNIT ( ) SI_UNIT ( $, .RADIAN. ) );
#11901=CARTESIAN_POINT ( 'NONE',  ( -828.3244535745621988, 80.88628718089528036, -154.4158655367039330 ) ) ;
#11902=CARTESIAN_POINT ( 'NONE',  ( -819.2376510598700179, 55.50059629688461627, -96.78565065507937959 ) ) ;
#11905=CARTESIAN_POINT ( 'NONE',  ( -991.5701548301635739, 122.8678427087061493, -126.6442663926292056 ) ) ;
#11912=CARTESIAN_POINT ( 'NONE',  ( -998.0431609429220998, 37.14019503514176535, -124.6807709998042668 ) ) ;
#11913=CARTESIAN_POINT ( 'NONE',  ( -818.8285638327253082, 78.34424586195346762, -154.6388909787697798 ) ) ;
#11917=CARTESIAN_POINT ( 'NONE',  ( -1045.864486809339724, 115.5688325305733741, -124.6807709998043663 ) ) ;
#11924=ORIENTED_EDGE ( 'NONE', *, *, #12205, .T. ) ;
#11925=CARTESIAN_POINT ( 'NONE',  ( -1065.000000000006594, 112.0000000000007105, -124.6807709998041531 ) ) ;
#11939=CARTESIAN_POINT ( 'NONE',  ( -818.6751755801125228, 47.70925804672287995, -149.7857175106634884 ) ) ;
#11949=VERTEX_POINT ( 'NONE', #5216 ) ;
#11951=CYLINDRICAL_SURFACE ( 'NONE', #3853, 5.000000000000115463 ) ;
#11956=CARTESIAN_POINT ( 'NONE',  ( -818.9903241194234624, 79.97817460710089676, -154.5468534023889049 ) ) ;
#11957=AXIS2_PLACEMENT_3D ( 'NONE', #9048, #10904, #7955 ) ;
#11958=CARTESIAN_POINT ( 'NONE',  ( -1015.825132819593136, 80.44428838836749662, -95.06748246948035330 ) ) ;
#11964=CARTESIAN_POINT ( 'NONE',  ( -822.0656543776474336, 83.35610039114051517, -154.1646031964236556 ) ) ;
#11981=CARTESIAN_POINT ( 'NONE',  ( -1010.922847972425529, 120.6260792194948550, -124.6807709998039542 ) ) ;
#11992=CARTESIAN_POINT ( 'NONE',  ( -903.2629211055218548, 97.63080833215174437, -154.2940595301276971 ) ) ;
#11995=DIRECTION ( 'NONE',  ( 0.000000000000000000, 1.000000000000000000, 6.938893903907169213E-16 ) ) ;
#11996=CARTESIAN_POINT ( 'NONE',  ( -952.4132309232853686, 101.5728619241206161, -152.5758913445289409 ) ) ;
#12002=CARTESIAN_POINT ( 'NONE',  ( -1016.123300349502756, 74.17810748283176281, -152.5758913445294525 ) ) ;
#12012=CARTESIAN_POINT ( 'NONE',  ( -1032.644706488202019, 45.21923725197559207, -130.5712005305405228 ) ) ;
#12017=CARTESIAN_POINT ( 'NONE',  ( -927.6556653799030983, 86.18751778479037284, -95.06748246948041015 ) ) ;
#12026=EDGE_LOOP ( 'NONE', ( #5938, #11785, #4809, #10959 ) ) ;
#12027=CARTESIAN_POINT ( 'NONE',  ( -823.5011947277521358, 83.67454157012906535, -154.1077669601579032 ) ) ;
#12028=CARTESIAN_POINT ( 'NONE',  ( -795.0000000000080718, 82.00000000000049738, -94.48732055948593711 ) ) ;
#12029=CARTESIAN_POINT ( 'NONE',  ( -795.0000000000043201, 82.00000000000039790, -124.6807709998041105 ) ) ;
#12031=CARTESIAN_POINT ( 'NONE',  ( -955.0000000000038654, 82.00000000000036948, -124.6807709998041673 ) ) ;
#12043=CARTESIAN_POINT ( 'NONE',  ( -823.8285638327243987, 78.67432280806571043, -264.6807709998050200 ) ) ;
#12044=CARTESIAN_POINT ( 'NONE',  ( -1021.743962174751232, 119.2557508373789403, -124.6807709998040110 ) ) ;
#12054=CARTESIAN_POINT ( 'NONE',  ( -1026.284439350006778, 91.37828661775253636, -154.2940595301281803 ) ) ;
#12058=CARTESIAN_POINT ( 'NONE',  ( -993.6119331254993767, 96.30709745136249467, -152.5758913445288840 ) ) ;
#12066=CARTESIAN_POINT ( 'NONE',  ( -1020.082665824768128, 80.34198733739798115, -154.2940595301280950 ) ) ;
#12087=CARTESIAN_POINT ( 'NONE',  ( -955.3297122972882107, 93.84065249268854814, -95.06748246948001224 ) ) ;
#12089=CARTESIAN_POINT ( 'NONE',  ( -957.2086549536783195, 47.65337959301152893, -126.6442663926291345 ) ) ;
#12098=CARTESIAN_POINT ( 'NONE',  ( -1021.046747802643722, 63.38047825189596551, -103.3307627799639761 ) ) ;
#12112=CARTESIAN_POINT ( 'NONE',  ( -1037.337636019038882, 116.9882293220588991, -124.6807709998043521 ) ) ;
#12122=CARTESIAN_POINT ( 'NONE',  ( -1037.337636019038882, 116.9882293220588991, -124.6807709998043521 ) ) ;
#12125=CARTESIAN_POINT ( 'NONE',  ( -853.3345817150077437, 81.97571759610561060, -154.2940595301280098 ) ) ;
#12135=CARTESIAN_POINT ( 'NONE',  ( -1047.626240907250804, 63.12837257276900260, -152.5758913445295093 ) ) ;
#12143=CARTESIAN_POINT ( 'NONE',  ( -827.6116171724385140, 75.38904402457046672, -105.8033998852344695 ) ) ;
#12156=CARTESIAN_POINT ( 'NONE',  ( -955.9230626098324137, 78.80814421416175719, -95.06748246948052383 ) ) ;
#12166=CARTESIAN_POINT ( 'NONE',  ( -1016.402231264574652, 68.39482517277133411, -99.57582448894554261 ) ) ;
#12169=DIRECTION ( 'NONE',  ( 0.000000000000000000, 1.000000000000000000, 6.938893903907169213E-16 ) ) ;
#12180=CARTESIAN_POINT ( 'NONE',  ( -904.0006525278403160, 119.6095687608906672, -107.9061927053323160 ) ) ;
#12186=CARTESIAN_POINT ( 'NONE',  ( -974.1288507787422759, 124.2142274477005657, -124.6807709998040110 ) ) ;
#12190=CARTESIAN_POINT ( 'NONE',  ( -952.6992609796615170, 94.45070821375009018, -154.2940595301278961 ) ) ;
#12193=CARTESIAN_POINT ( 'NONE',  ( -1046.676250823071769, 92.10743237175765330, -152.5758913445291967 ) ) ;
#12197=CARTESIAN_POINT ( 'NONE',  ( -795.0000000000071623, 70.44548139156209743, -152.5758913445292535 ) ) ;
#12201=CARTESIAN_POINT ( 'NONE',  ( -828.0828412852945348, 81.30646073758887837, -144.6692115456662862 ) ) ;
#12205=EDGE_CURVE ( 'NONE', #11269, #4723, #1616, .T. ) ;
#12212=CARTESIAN_POINT ( 'NONE',  ( -902.6139906877451722, 77.75433758651645633, -96.78565065507919485 ) ) ;
#12213=CARTESIAN_POINT ( 'NONE',  ( -824.4866663711965202, 83.64159454339613831, -104.7481522953016224 ) ) ;
#12214=CARTESIAN_POINT ( 'NONE',  ( -854.0902776497797504, 23.28889115110667518, -126.6442663926296603 ) ) ;
#12215=CARTESIAN_POINT ( 'NONE',  ( -822.5351658412997722, 83.51517767605579934, -144.6233963009600529 ) ) ;
#12221=CARTESIAN_POINT ( 'NONE',  ( -1038.506348936316726, 51.71309463382168303, -103.3307627799636350 ) ) ;
#12223=DIRECTION ( 'NONE',  ( 0.000000000000000000, 5.522905491341382306E-16, 1.000000000000000000 ) ) ;
#12224=B_SPLINE_CURVE_WITH_KNOTS ( 'NONE', 3,
 ( #1588, #11913, #5484, #8216, #3433, #7281, #11049, #7219, #5350, #2574, #10597, #9728, #3926, #11714, #7820, #7005, #385, #2312, #3112, #8692, #326, #9672, #142, #1266, #11653, #9609, #3056, #1211, #4112, #6759, #8804, #1091, #202, #8628, #3986, #10716, #7696, #7941, #10777, #4166 ),
 .UNSPECIFIED., .F., .F.,
 ( 4, 2, 2, 2, 2, 2, 2, 2, 2, 2, 2, 2, 2, 2, 2, 2, 2, 2, 2, 4 ),
 ( 6.938893903908117079E-17, 0.0009772159915550746208, 0.001465823987332597837, 0.001954431983110120619, 0.002931647974665001818, 0.003908863966219883017, 0.004886079957774763782, 0.005863295949329645415, 0.006840511940884527048, 0.007817727932439406946, 0.008794943923994288579, 0.009772159915549170212, 0.01026076791132677322, 0.01074937590710437277, 0.01172659189865929950, 0.01270380789021422624, 0.01319241588599166966, 0.01368102388176911655, 0.01465823987332400859, 0.01563545586487890063 ),
 .UNSPECIFIED. ) ;
#12230=CARTESIAN_POINT ( 'NONE',  ( -795.0000000000002274, 107.1049510380560719, -107.9061927053326002 ) ) ;
#12237=CARTESIAN_POINT ( 'NONE',  ( -1024.848917040348397, 116.4131098345821442, -113.1262384684097242 ) ) ;
#12239=CARTESIAN_POINT ( 'NONE',  ( -994.8066578865465317, 80.00401887192411721, -154.8742214401228523 ) ) ;
ENDSEC;
END-ISO-10303-21;
